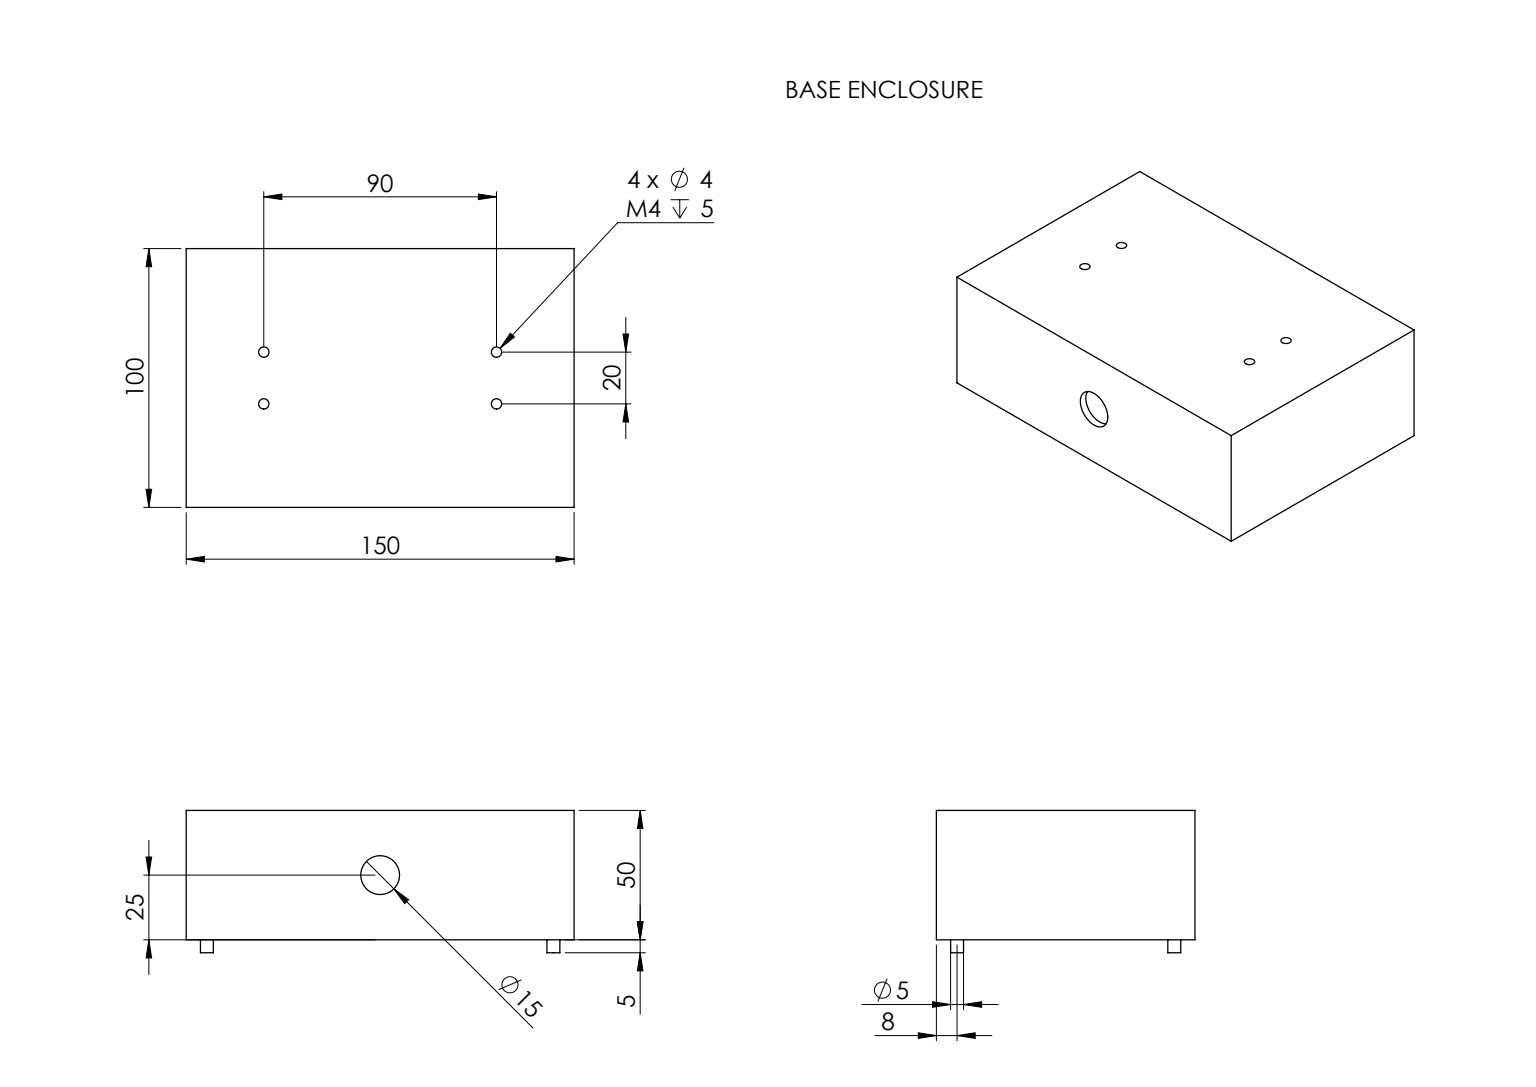
ISO-10303-21;
HEADER;
FILE_DESCRIPTION (('STEP AP214'),
    '1' );
FILE_NAME ('Base Enclosure^MAS-192.step',
    '2026-10-24T04:45:50',
    ( '' ),
    ( '' ),
    'SwSTEP 2.0',
    'SolidWorks 2026',
    '' );
FILE_SCHEMA (( 'AUTOMOTIVE_DESIGN' ));
ENDSEC;

DATA;
#4=ORIENTED_EDGE ( 'NONE', *, *, #1160, .F. ) ;
#11=FACE_OUTER_BOUND ( 'NONE', #1438, .T. ) ;
#19=CARTESIAN_POINT ( 'NONE',  ( 66.99999999999997158, -5.000000000000000000, -44.49999999999999289 ) ) ;
#24=EDGE_CURVE ( 'NONE', #3154, #2478, #414, .T. ) ;
#26=ORIENTED_EDGE ( 'NONE', *, *, #2595, .T. ) ;
#32=EDGE_CURVE ( 'NONE', #3203, #1539, #250, .T. ) ;
#35=VERTEX_POINT ( 'NONE', #2248 ) ;
#39=DIRECTION ( 'NONE',  ( -0.000000000000000000, 1.000000000000000000, -0.000000000000000000 ) ) ;
#41=ORIENTED_EDGE ( 'NONE', *, *, #2652, .T. ) ;
#43=EDGE_CURVE ( 'NONE', #2320, #2585, #1939, .T. ) ;
#48=FACE_OUTER_BOUND ( 'NONE', #483, .T. ) ;
#50=CYLINDRICAL_SURFACE ( 'NONE', #2706, 2.000000000000001776 ) ;
#51=CIRCLE ( 'NONE', #1902, 2.000000000000001776 ) ;
#55=AXIS2_PLACEMENT_3D ( 'NONE', #952, #3052, #3261 ) ;
#58=DIRECTION ( 'NONE',  ( -0.000000000000000000, 1.000000000000000000, -0.000000000000000000 ) ) ;
#62=CARTESIAN_POINT ( 'NONE',  ( 75.00000000000000000, 0.000000000000000000, 50.00000000000000000 ) ) ;
#65=CARTESIAN_POINT ( 'NONE',  ( 44.99999999999999289, 50.00000000000000000, -10.00000000000000533 ) ) ;
#66=PRODUCT_DEFINITION ( 'UNKNOWN', '', #1367, #996 ) ;
#70=ORIENTED_EDGE ( 'NONE', *, *, #2599, .T. ) ;
#72=LINE ( 'NONE', #1928, #2609 ) ;
#76=ADVANCED_FACE ( 'NONE', ( #408 ), #1739, .F. ) ;
#77=UNCERTAINTY_MEASURE_WITH_UNIT (LENGTH_MEASURE( 1.000000000000000082E-05 ), #1447, 'distance_accuracy_value', 'NONE');
#81=DIRECTION ( 'NONE',  ( 0.000000000000000000, 0.000000000000000000, -1.000000000000000000 ) ) ;
#82=LINE ( 'NONE', #1653, #2818 ) ;
#87=DIRECTION ( 'NONE',  ( 0.000000000000000000, 0.000000000000000000, 1.000000000000000000 ) ) ;
#88=ORIENTED_EDGE ( 'NONE', *, *, #1626, .T. ) ;
#92=DIRECTION ( 'NONE',  ( 0.000000000000000000, 0.000000000000000000, 1.000000000000000000 ) ) ;
#93=ADVANCED_FACE ( 'NONE', ( #3005 ), #3282, .F. ) ;
#94=CIRCLE ( 'NONE', #1191, 2.499999999999995115 ) ;
#96=CARTESIAN_POINT ( 'NONE',  ( -74.99999999999998579, 50.00000000000000000, -50.00000000000000000 ) ) ;
#97=AXIS2_PLACEMENT_3D ( 'NONE', #437, #2770, #128 ) ;
#103=FACE_BOUND ( 'NONE', #1561, .T. ) ;
#113=VERTEX_POINT ( 'NONE', #494 ) ;
#115=CARTESIAN_POINT ( 'NONE',  ( 66.99999999999997158, -5.000000000000000000, -39.50000000000000000 ) ) ;
#118=ADVANCED_FACE ( 'NONE', ( #1534 ), #3208, .F. ) ;
#119=CARTESIAN_POINT ( 'NONE',  ( -74.99999999999998579, 50.00000000000000000, -50.00000000000000000 ) ) ;
#121=VERTEX_POINT ( 'NONE', #1820 ) ;
#122=FACE_BOUND ( 'NONE', #2327, .T. ) ;
#123=FACE_OUTER_BOUND ( 'NONE', #1619, .T. ) ;
#125=LINE ( 'NONE', #3241, #2277 ) ;
#126=PRODUCT_CONTEXT ( 'NONE', #916, 'mechanical' ) ;
#128=DIRECTION ( 'NONE',  ( 1.000000000000000000, 0.000000000000000000, 0.000000000000000000 ) ) ;
#132=CARTESIAN_POINT ( 'NONE',  ( -66.99999999999997158, 0.000000000000000000, -41.99999999999999289 ) ) ;
#133=EDGE_CURVE ( 'NONE', #3190, #3154, #2535, .T. ) ;
#134=CARTESIAN_POINT ( 'NONE',  ( 0.000000000000000000, 25.00000000000000000, 50.00000000000000000 ) ) ;
#142=ORIENTED_EDGE ( 'NONE', *, *, #43, .F. ) ;
#148=DIRECTION ( 'NONE',  ( -0.000000000000000000, 1.000000000000000000, -0.000000000000000000 ) ) ;
#158=CIRCLE ( 'NONE', #2772, 2.499999999999995115 ) ;
#170=CARTESIAN_POINT ( 'NONE',  ( -75.00000000000000000, 50.00000000000000000, 50.00000000000000000 ) ) ;
#172=DIRECTION ( 'NONE',  ( 0.000000000000000000, 0.000000000000000000, -1.000000000000000000 ) ) ;
#173=EDGE_LOOP ( 'NONE', ( #2677, #3008, #1781, #962 ) ) ;
#176=ORIENTED_EDGE ( 'NONE', *, *, #433, .T. ) ;
#178=CARTESIAN_POINT ( 'NONE',  ( 44.99999999999999289, 50.00000000000000000, -12.00000000000000711 ) ) ;
#180=ORIENTED_EDGE ( 'NONE', *, *, #1149, .T. ) ;
#183=DIRECTION ( 'NONE',  ( -0.000000000000000000, 1.000000000000000000, -0.000000000000000000 ) ) ;
#185=DIRECTION ( 'NONE',  ( -0.000000000000000000, 1.000000000000000000, 0.000000000000000000 ) ) ;
#186=CARTESIAN_POINT ( 'NONE',  ( -66.99999999999997158, -5.000000000000000000, -41.99999999999999289 ) ) ;
#191=CARTESIAN_POINT ( 'NONE',  ( -45.00000000000000000, 43.79827876194489278, -9.999999999999994671 ) ) ;
#192=ORIENTED_EDGE ( 'NONE', *, *, #815, .F. ) ;
#203=ORIENTED_EDGE ( 'NONE', *, *, #133, .F. ) ;
#206=AXIS2_PLACEMENT_3D ( 'NONE', #944, #2253, #978 ) ;
#208=ORIENTED_EDGE ( 'NONE', *, *, #1510, .T. ) ;
#209=CIRCLE ( 'NONE', #2120, 2.499999999999995115 ) ;
#213=VECTOR ( 'NONE', #1718, 1000.000000000000000 ) ;
#226=ORIENTED_EDGE ( 'NONE', *, *, #721, .T. ) ;
#227=CARTESIAN_POINT ( 'NONE',  ( 7.500000000000000000, 25.00000000000000000, 50.00000000000000000 ) ) ;
#232=CARTESIAN_POINT ( 'NONE',  ( 45.00000000000000000, 50.00000000000000000, 9.999999999999994671 ) ) ;
#234=CARTESIAN_POINT ( 'NONE',  ( 66.99999999999997158, 0.000000000000000000, -41.99999999999999289 ) ) ;
#238=ORIENTED_EDGE ( 'NONE', *, *, #3134, .T. ) ;
#246=CARTESIAN_POINT ( 'NONE',  ( -44.99999999999999289, 45.00000000000000711, 12.00000000000000711 ) ) ;
#248=EDGE_CURVE ( 'NONE', #1538, #561, #458, .T. ) ;
#250=CIRCLE ( 'NONE', #2594, 2.000000000000001776 ) ;
#252=DIRECTION ( 'NONE',  ( 0.000000000000000000, 0.000000000000000000, 1.000000000000000000 ) ) ;
#263=AXIS2_PLACEMENT_3D ( 'NONE', #2360, #1555, #2633 ) ;
#264=ORIENTED_EDGE ( 'NONE', *, *, #1320, .T. ) ;
#267=DIRECTION ( 'NONE',  ( -0.000000000000000000, -1.000000000000000000, -0.000000000000000000 ) ) ;
#270=CYLINDRICAL_SURFACE ( 'NONE', #435, 2.000000000000001776 ) ;
#277=VERTEX_POINT ( 'NONE', #2558 ) ;
#279=AXIS2_PLACEMENT_3D ( 'NONE', #1513, #2605, #2846 ) ;
#282=DIRECTION ( 'NONE',  ( -1.000000000000000000, 0.000000000000000000, 0.000000000000000000 ) ) ;
#283=EDGE_CURVE ( 'NONE', #2585, #480, #1268, .T. ) ;
#286=CARTESIAN_POINT ( 'NONE',  ( 75.00000000000000000, 50.00000000000000000, 50.00000000000000000 ) ) ;
#290=DIRECTION ( 'NONE',  ( -0.000000000000000000, 1.000000000000000000, -0.000000000000000000 ) ) ;
#292=ORIENTED_EDGE ( 'NONE', *, *, #3182, .F. ) ;
#294=CYLINDRICAL_SURFACE ( 'NONE', #263, 2.000000000000001776 ) ;
#298=CYLINDRICAL_SURFACE ( 'NONE', #3325, 2.499999999999995115 ) ;
#300=DIRECTION ( 'NONE',  ( -0.000000000000000000, 1.000000000000000000, -0.000000000000000000 ) ) ;
#301=SURFACE_STYLE_USAGE ( .BOTH. , #1377 ) ;
#302=FACE_BOUND ( 'NONE', #1880, .T. ) ;
#307=ORIENTED_EDGE ( 'NONE', *, *, #2205, .T. ) ;
#308=LINE ( 'NONE', #1347, #2939 ) ;
#310=EDGE_CURVE ( 'NONE', #2398, #468, #2110, .T. ) ;
#314=AXIS2_PLACEMENT_3D ( 'NONE', #1704, #183, #1430 ) ;
#320=AXIS2_PLACEMENT_3D ( 'NONE', #3066, #1000, #486 ) ;
#323=CARTESIAN_POINT ( 'NONE',  ( 45.00000000000000000, 45.00000000000000711, 7.999999999999992895 ) ) ;
#324=VECTOR ( 'NONE', #1168, 999.9999999999998863 ) ;
#325=EDGE_CURVE ( 'NONE', #1539, #3203, #1947, .T. ) ;
#330=CYLINDRICAL_SURFACE ( 'NONE', #1898, 2.000000000000001776 ) ;
#332=LINE ( 'NONE', #2410, #1914 ) ;
#333=( LENGTH_UNIT ( ) NAMED_UNIT ( * ) SI_UNIT ( .MILLI., .METRE. ) );
#341=ORIENTED_EDGE ( 'NONE', *, *, #1510, .F. ) ;
#345=ORIENTED_EDGE ( 'NONE', *, *, #1998, .T. ) ;
#347=VERTEX_POINT ( 'NONE', #3209 ) ;
#350=DIRECTION ( 'NONE',  ( -0.000000000000000000, 1.000000000000000000, -0.000000000000000000 ) ) ;
#362=ADVANCED_FACE ( 'NONE', ( #830 ), #478, .F. ) ;
#368=DIRECTION ( 'NONE',  ( 0.000000000000000000, 0.000000000000000000, 1.000000000000000000 ) ) ;
#369=VECTOR ( 'NONE', #2367, 1000.000000000000000 ) ;
#372=ORIENTED_EDGE ( 'NONE', *, *, #3079, .F. ) ;
#375=CIRCLE ( 'NONE', #1306, 2.499999999999995115 ) ;
#376=ORIENTED_EDGE ( 'NONE', *, *, #1556, .T. ) ;
#377=FACE_BOUND ( 'NONE', #2636, .T. ) ;
#381=ORIENTED_EDGE ( 'NONE', *, *, #248, .F. ) ;
#382=CIRCLE ( 'NONE', #279, 2.499999999999995115 ) ;
#393=FACE_OUTER_BOUND ( 'NONE', #821, .T. ) ;
#400=ADVANCED_FACE ( 'NONE', ( #302, #1340 ), #2369, .F. ) ;
#402=ORIENTED_EDGE ( 'NONE', *, *, #3206, .F. ) ;
#403=CARTESIAN_POINT ( 'NONE',  ( 66.99999999999997158, -5.000000000000000000, -41.99999999999999289 ) ) ;
#407=CARTESIAN_POINT ( 'NONE',  ( -45.00000000000000000, 50.00000000000000000, -7.999999999999992895 ) ) ;
#408=FACE_OUTER_BOUND ( 'NONE', #1187, .T. ) ;
#411=ORIENTED_EDGE ( 'NONE', *, *, #2806, .T. ) ;
#414=CIRCLE ( 'NONE', #849, 7.500000000000000000 ) ;
#420=DIRECTION ( 'NONE',  ( 0.000000000000000000, -1.000000000000000000, 0.000000000000000000 ) ) ;
#421=CARTESIAN_POINT ( 'NONE',  ( -45.00000000000000000, 50.00000000000000000, -9.999999999999994671 ) ) ;
#423=DIRECTION ( 'NONE',  ( 0.000000000000000000, -1.000000000000000000, 0.000000000000000000 ) ) ;
#424=AXIS2_PLACEMENT_3D ( 'NONE', #2897, #2673, #1362 ) ;
#425=ADVANCED_FACE ( 'NONE', ( #48 ), #847, .T. ) ;
#426=( NAMED_UNIT ( * ) SI_UNIT ( $, .STERADIAN. ) SOLID_ANGLE_UNIT ( ) );
#427=AXIS2_PLACEMENT_3D ( 'NONE', #2477, #1108, #87 ) ;
#429=ORIENTED_EDGE ( 'NONE', *, *, #1320, .F. ) ;
#432=VECTOR ( 'NONE', #2012, 999.9999999999998863 ) ;
#433=EDGE_CURVE ( 'NONE', #2761, #2259, #1907, .T. ) ;
#435=AXIS2_PLACEMENT_3D ( 'NONE', #232, #1280, #3107 ) ;
#437=CARTESIAN_POINT ( 'NONE',  ( 0.000000000000000000, 25.00000000000000000, 47.00000000000000000 ) ) ;
#443=EDGE_CURVE ( 'NONE', #277, #2259, #3036, .T. ) ;
#444=DIRECTION ( 'NONE',  ( -0.000000000000000000, 1.000000000000000000, -0.000000000000000000 ) ) ;
#448=VERTEX_POINT ( 'NONE', #2198 ) ;
#453=PLANE ( 'NONE',  #2663 ) ;
#454=ORIENTED_EDGE ( 'NONE', *, *, #1869, .T. ) ;
#458=LINE ( 'NONE', #1514, #910 ) ;
#460=LINE ( 'NONE', #3299, #3221 ) ;
#461=ORIENTED_EDGE ( 'NONE', *, *, #1991, .F. ) ;
#463=CARTESIAN_POINT ( 'NONE',  ( -66.99999999999997158, -5.000000000000000000, 39.50000000000000000 ) ) ;
#466=PLANE ( 'NONE',  #320 ) ;
#468=VERTEX_POINT ( 'NONE', #1178 ) ;
#470=DIRECTION ( 'NONE',  ( 1.049727191138620668E-16, 0.5150380749100514910, -0.8571673007021138879 ) ) ;
#473=CARTESIAN_POINT ( 'NONE',  ( -45.00000000000000000, 50.00000000000000000, -9.999999999999994671 ) ) ;
#478=CONICAL_SURFACE ( 'NONE', #424, 2.000000000000001776, 1.029744258676657642 ) ;
#479=ADVANCED_BREP_SHAPE_REPRESENTATION ( '', ( #2792, #3111 ), #1204 ) ;
#480=VERTEX_POINT ( 'NONE', #2212 ) ;
#483=EDGE_LOOP ( 'NONE', ( #402, #2152, #70, #1488 ) ) ;
#486=DIRECTION ( 'NONE',  ( 0.000000000000000000, -0.000000000000000000, -1.000000000000000000 ) ) ;
#492=ADVANCED_FACE ( 'NONE', ( #3247 ), #1936, .F. ) ;
#494=CARTESIAN_POINT ( 'NONE',  ( 44.99999999999999289, 45.00000000000000711, -8.000000000000003553 ) ) ;
#495=CARTESIAN_POINT ( 'NONE',  ( 75.00000000000000000, 0.000000000000000000, -50.00000000000000000 ) ) ;
#498=ORIENTED_EDGE ( 'NONE', *, *, #1764, .F. ) ;
#499=VERTEX_POINT ( 'NONE', #1703 ) ;
#504=DIRECTION ( 'NONE',  ( 0.000000000000000000, 0.000000000000000000, 1.000000000000000000 ) ) ;
#507=FACE_OUTER_BOUND ( 'NONE', #752, .T. ) ;
#510=PRODUCT ( 'Base Enclosure^MAS-192', 'Base Enclosure^MAS-192', '', ( #126 ) ) ;
#511=EDGE_CURVE ( 'NONE', #1605, #1554, #94, .T. ) ;
#515=EDGE_LOOP ( 'NONE', ( #3254, #1310, #3355, #3169 ) ) ;
#520=DIRECTION ( 'NONE',  ( -0.000000000000000000, 1.000000000000000000, -0.000000000000000000 ) ) ;
#523=LINE ( 'NONE', #2574, #1629 ) ;
#531=VERTEX_POINT ( 'NONE', #2484 ) ;
#532=AXIS2_PLACEMENT_3D ( 'NONE', #403, #2962, #671 ) ;
#537=CIRCLE ( 'NONE', #3045, 2.000000000000001776 ) ;
#548=ORIENTED_EDGE ( 'NONE', *, *, #3058, .T. ) ;
#551=ORIENTED_EDGE ( 'NONE', *, *, #1747, .F. ) ;
#552=DIRECTION ( 'NONE',  ( 0.000000000000000000, 0.000000000000000000, 1.000000000000000000 ) ) ;
#553=UNCERTAINTY_MEASURE_WITH_UNIT (LENGTH_MEASURE( 1.000000000000000082E-05 ), #1906, 'distance_accuracy_value', 'NONE');
#557=CARTESIAN_POINT ( 'NONE',  ( 45.00000000000000000, 45.00000000000000711, 9.999999999999994671 ) ) ;
#561=VERTEX_POINT ( 'NONE', #1479 ) ;
#562=ORIENTED_EDGE ( 'NONE', *, *, #1667, .F. ) ;
#564=ORIENTED_EDGE ( 'NONE', *, *, #2324, .F. ) ;
#569=DIRECTION ( 'NONE',  ( -0.000000000000000000, 1.000000000000000000, -0.000000000000000000 ) ) ;
#577=FACE_OUTER_BOUND ( 'NONE', #3185, .T. ) ;
#584=AXIS2_PLACEMENT_3D ( 'NONE', #1266, #520, #989 ) ;
#590=DIRECTION ( 'NONE',  ( 0.000000000000000000, 0.000000000000000000, 1.000000000000000000 ) ) ;
#594=VERTEX_POINT ( 'NONE', #2044 ) ;
#597=CARTESIAN_POINT ( 'NONE',  ( -44.99999999999999289, 45.00000000000000711, 10.00000000000000533 ) ) ;
#598=DIRECTION ( 'NONE',  ( 1.000000000000000000, -0.000000000000000000, 1.387778780781445676E-16 ) ) ;
#603=EDGE_CURVE ( 'NONE', #448, #2691, #764, .T. ) ;
#609=ORIENTED_EDGE ( 'NONE', *, *, #721, .F. ) ;
#611=EDGE_CURVE ( 'NONE', #2086, #347, #1767, .T. ) ;
#618=CARTESIAN_POINT ( 'NONE',  ( -45.00000000000000000, 50.00000000000000000, -11.99999999999999645 ) ) ;
#620=PRESENTATION_STYLE_ASSIGNMENT (( #301 ) ) ;
#623=FACE_OUTER_BOUND ( 'NONE', #2591, .T. ) ;
#626=DIRECTION ( 'NONE',  ( -0.000000000000000000, 1.000000000000000000, -0.000000000000000000 ) ) ;
#630=EDGE_CURVE ( 'NONE', #347, #2291, #3348, .T. ) ;
#633=ADVANCED_FACE ( 'NONE', ( #781 ), #2027, .F. ) ;
#642=CARTESIAN_POINT ( 'NONE',  ( -66.99999999999997158, -5.000000000000000000, 44.49999999999999289 ) ) ;
#645=DIRECTION ( 'NONE',  ( -0.000000000000000000, 1.000000000000000000, -0.000000000000000000 ) ) ;
#646=EDGE_CURVE ( 'NONE', #2761, #113, #2061, .T. ) ;
#651=EDGE_LOOP ( 'NONE', ( #1357, #2209 ) ) ;
#655=ORIENTED_EDGE ( 'NONE', *, *, #3079, .T. ) ;
#656=CARTESIAN_POINT ( 'NONE',  ( 44.99999999999999289, 45.00000000000000711, -12.00000000000000711 ) ) ;
#657=DIRECTION ( 'NONE',  ( 0.000000000000000000, 0.000000000000000000, 1.000000000000000000 ) ) ;
#660=DIRECTION ( 'NONE',  ( 1.000000000000000000, 0.000000000000000000, 0.000000000000000000 ) ) ;
#661=CYLINDRICAL_SURFACE ( 'NONE', #314, 2.499999999999995115 ) ;
#663=DIRECTION ( 'NONE',  ( 0.000000000000000000, 0.000000000000000000, 1.000000000000000000 ) ) ;
#671=DIRECTION ( 'NONE',  ( 0.000000000000000000, -0.000000000000000000, -1.000000000000000000 ) ) ;
#672=CARTESIAN_POINT ( 'NONE',  ( 66.99999999999997158, -5.000000000000000000, -41.99999999999999289 ) ) ;
#673=FACE_OUTER_BOUND ( 'NONE', #3258, .T. ) ;
#678=( NAMED_UNIT ( * ) PLANE_ANGLE_UNIT ( ) SI_UNIT ( $, .RADIAN. ) );
#679=ORIENTED_EDGE ( 'NONE', *, *, #3237, .T. ) ;
#685=SHAPE_REPRESENTATION ( 'Base Enclosure^MAS-192', ( #3111 ), #1204 ) ;
#690=CARTESIAN_POINT ( 'NONE',  ( -7.500000000000000000, 25.00000000000000000, 47.00000000000000000 ) ) ;
#695=AXIS2_PLACEMENT_3D ( 'NONE', #1058, #2991, #2351 ) ;
#696=DIRECTION ( 'NONE',  ( 0.000000000000000000, 0.000000000000000000, 1.000000000000000000 ) ) ;
#700=DIRECTION ( 'NONE',  ( -0.000000000000000000, 1.000000000000000000, 0.000000000000000000 ) ) ;
#702=CIRCLE ( 'NONE', #1036, 2.499999999999995115 ) ;
#709=ORIENTED_EDGE ( 'NONE', *, *, #2219, .T. ) ;
#719=VERTEX_POINT ( 'NONE', #2682 ) ;
#721=EDGE_CURVE ( 'NONE', #468, #3203, #2942, .T. ) ;
#728=LINE ( 'NONE', #1509, #1455 ) ;
#731=CARTESIAN_POINT ( 'NONE',  ( -66.99999999999997158, 0.000000000000000000, 41.99999999999999289 ) ) ;
#733=ORIENTED_EDGE ( 'NONE', *, *, #3213, .T. ) ;
#735=ORIENTED_EDGE ( 'NONE', *, *, #2411, .F. ) ;
#737=DIRECTION ( 'NONE',  ( 0.000000000000000000, -1.000000000000000000, 0.000000000000000000 ) ) ;
#748=ORIENTED_EDGE ( 'NONE', *, *, #283, .T. ) ;
#752=EDGE_LOOP ( 'NONE', ( #2089, #1877, #2801, #609 ) ) ;
#757=AXIS2_PLACEMENT_3D ( 'NONE', #1609, #2090, #2144 ) ;
#758=CIRCLE ( 'NONE', #2664, 2.499999999999995115 ) ;
#763=ORIENTED_EDGE ( 'NONE', *, *, #1960, .F. ) ;
#764=LINE ( 'NONE', #2586, #2546 ) ;
#768=CARTESIAN_POINT ( 'NONE',  ( -45.00000000000000000, 45.00000000000000711, -9.999999999999994671 ) ) ;
#771=PLANE ( 'NONE',  #2227 ) ;
#774=VERTEX_POINT ( 'NONE', #2712 ) ;
#777=EDGE_CURVE ( 'NONE', #3174, #895, #2769, .T. ) ;
#781=FACE_OUTER_BOUND ( 'NONE', #515, .T. ) ;
#791=EDGE_LOOP ( 'NONE', ( #1449, #2166, #1868, #3198 ) ) ;
#792=LINE ( 'NONE', #1337, #2392 ) ;
#798=CARTESIAN_POINT ( 'NONE',  ( 0.000000000000000000, 25.00000000000000000, 47.00000000000000000 ) ) ;
#801=VERTEX_POINT ( 'NONE', #857 ) ;
#805=AXIS2_PLACEMENT_3D ( 'NONE', #2415, #865, #2687 ) ;
#806=ORIENTED_EDGE ( 'NONE', *, *, #2411, .T. ) ;
#809=CIRCLE ( 'NONE', #2548, 2.000000000000001776 ) ;
#811=AXIS2_PLACEMENT_3D ( 'NONE', #2678, #2903, #1154 ) ;
#812=ORIENTED_EDGE ( 'NONE', *, *, #2257, .F. ) ;
#813=FACE_OUTER_BOUND ( 'NONE', #173, .T. ) ;
#815=EDGE_CURVE ( 'NONE', #561, #719, #125, .T. ) ;
#817=CARTESIAN_POINT ( 'NONE',  ( 75.00000000000000000, 50.00000000000000000, 50.00000000000000000 ) ) ;
#818=DIRECTION ( 'NONE',  ( 0.000000000000000000, 0.000000000000000000, 1.000000000000000000 ) ) ;
#821=EDGE_LOOP ( 'NONE', ( #1255, #1521, #1611, #3308 ) ) ;
#824=VERTEX_POINT ( 'NONE', #1932 ) ;
#826=CYLINDRICAL_SURFACE ( 'NONE', #3105, 2.499999999999995115 ) ;
#828=ORIENTED_EDGE ( 'NONE', *, *, #1481, .T. ) ;
#830=FACE_OUTER_BOUND ( 'NONE', #2341, .T. ) ;
#832=DIRECTION ( 'NONE',  ( -0.000000000000000000, 1.000000000000000000, -0.000000000000000000 ) ) ;
#835=ORIENTED_EDGE ( 'NONE', *, *, #511, .F. ) ;
#837=FACE_OUTER_BOUND ( 'NONE', #1826, .T. ) ;
#842=EDGE_CURVE ( 'NONE', #1605, #1570, #332, .T. ) ;
#847=CYLINDRICAL_SURFACE ( 'NONE', #805, 2.499999999999995115 ) ;
#848=CARTESIAN_POINT ( 'NONE',  ( -45.00000000000000000, 50.00000000000000000, -9.999999999999994671 ) ) ;
#849=AXIS2_PLACEMENT_3D ( 'NONE', #134, #663, #1707 ) ;
#857=CARTESIAN_POINT ( 'NONE',  ( -44.99999999999999289, 50.00000000000000000, 8.000000000000003553 ) ) ;
#861=AXIS2_PLACEMENT_3D ( 'NONE', #1652, #290, #1635 ) ;
#864=SURFACE_STYLE_FILL_AREA ( #3179 ) ;
#865=DIRECTION ( 'NONE',  ( -0.000000000000000000, 1.000000000000000000, -0.000000000000000000 ) ) ;
#875=DIRECTION ( 'NONE',  ( 0.000000000000000000, 0.000000000000000000, 1.000000000000000000 ) ) ;
#876=DIRECTION ( 'NONE',  ( 0.000000000000000000, 0.5150380749100514910, 0.8571673007021138879 ) ) ;
#883=DIRECTION ( 'NONE',  ( -0.000000000000000000, -0.000000000000000000, 1.000000000000000000 ) ) ;
#884=DIRECTION ( 'NONE',  ( -0.000000000000000000, 1.000000000000000000, -0.000000000000000000 ) ) ;
#888=ORIENTED_EDGE ( 'NONE', *, *, #2262, .T. ) ;
#891=EDGE_CURVE ( 'NONE', #1277, #3215, #1450, .T. ) ;
#893=DIRECTION ( 'NONE',  ( -0.000000000000000000, 1.000000000000000000, -0.000000000000000000 ) ) ;
#895=VERTEX_POINT ( 'NONE', #463 ) ;
#910=VECTOR ( 'NONE', #1496, 1000.000000000000000 ) ;
#913=AXIS2_PLACEMENT_3D ( 'NONE', #3141, #2879, #1165 ) ;
#916=APPLICATION_CONTEXT ( 'automotive_design' ) ;
#917=CIRCLE ( 'NONE', #1141, 7.500000000000000000 ) ;
#921=VECTOR ( 'NONE', #3175, 1000.000000000000000 ) ;
#933=ORIENTED_EDGE ( 'NONE', *, *, #283, .F. ) ;
#937=CARTESIAN_POINT ( 'NONE',  ( 0.000000000000000000, 25.00000000000000000, 47.00000000000000000 ) ) ;
#939=DIRECTION ( 'NONE',  ( -0.000000000000000000, 1.000000000000000000, -0.000000000000000000 ) ) ;
#944=CARTESIAN_POINT ( 'NONE',  ( 66.99999999999997158, -5.000000000000000000, 41.99999999999999289 ) ) ;
#950=ORIENTED_EDGE ( 'NONE', *, *, #1226, .F. ) ;
#951=DIRECTION ( 'NONE',  ( 0.000000000000000000, -1.000000000000000000, 0.000000000000000000 ) ) ;
#952=CARTESIAN_POINT ( 'NONE',  ( 66.99999999999997158, 0.000000000000000000, 41.99999999999999289 ) ) ;
#953=ADVANCED_FACE ( 'NONE', ( #2745 ), #2269, .T. ) ;
#954=LINE ( 'NONE', #1988, #1308 ) ;
#956=CARTESIAN_POINT ( 'NONE',  ( 45.00000000000000000, 45.00000000000000711, 7.999999999999992895 ) ) ;
#962=ORIENTED_EDGE ( 'NONE', *, *, #1226, .T. ) ;
#965=AXIS2_PLACEMENT_3D ( 'NONE', #3127, #3072, #1786 ) ;
#968=LINE ( 'NONE', #2315, #981 ) ;
#970=EDGE_CURVE ( 'NONE', #2106, #1968, #809, .T. ) ;
#978=DIRECTION ( 'NONE',  ( 0.000000000000000000, 0.000000000000000000, 1.000000000000000000 ) ) ;
#980=CIRCLE ( 'NONE', #2557, 2.499999999999995115 ) ;
#981=VECTOR ( 'NONE', #1533, 1000.000000000000000 ) ;
#982=EDGE_LOOP ( 'NONE', ( #2278, #548, #2419 ) ) ;
#984=FACE_BOUND ( 'NONE', #1823, .T. ) ;
#989=DIRECTION ( 'NONE',  ( 0.000000000000000000, 0.000000000000000000, 1.000000000000000000 ) ) ;
#991=FACE_OUTER_BOUND ( 'NONE', #1558, .T. ) ;
#992=ADVANCED_FACE ( 'NONE', ( #1471 ), #3303, .F. ) ;
#996=PRODUCT_DEFINITION_CONTEXT ( 'detailed design', #2030, 'design' ) ;
#999=ORIENTED_EDGE ( 'NONE', *, *, #24, .F. ) ;
#1000=DIRECTION ( 'NONE',  ( 0.000000000000000000, -1.000000000000000000, 0.000000000000000000 ) ) ;
#1004=ADVANCED_FACE ( 'NONE', ( #3132 ), #294, .F. ) ;
#1007=DIRECTION ( 'NONE',  ( 0.000000000000000000, 0.000000000000000000, 1.000000000000000000 ) ) ;
#1010=ORIENTED_EDGE ( 'NONE', *, *, #2997, .F. ) ;
#1025=ORIENTED_EDGE ( 'NONE', *, *, #2262, .F. ) ;
#1026=VECTOR ( 'NONE', #1683, 1000.000000000000000 ) ;
#1027=VECTOR ( 'NONE', #876, 999.9999999999998863 ) ;
#1036=AXIS2_PLACEMENT_3D ( 'NONE', #186, #423, #3006 ) ;
#1038=UNCERTAINTY_MEASURE_WITH_UNIT (LENGTH_MEASURE( 1.000000000000000082E-05 ), #333, 'distance_accuracy_value', 'NONE');
#1046=DIRECTION ( 'NONE',  ( -0.000000000000000000, 1.000000000000000000, -0.000000000000000000 ) ) ;
#1055=CARTESIAN_POINT ( 'NONE',  ( 75.00000000000000000, 50.00000000000000000, 50.00000000000000000 ) ) ;
#1058=CARTESIAN_POINT ( 'NONE',  ( -66.99999999999997158, -5.000000000000000000, 41.99999999999999289 ) ) ;
#1069=DIRECTION ( 'NONE',  ( 0.000000000000000000, 0.000000000000000000, -1.000000000000000000 ) ) ;
#1078=LINE ( 'NONE', #2111, #2438 ) ;
#1086=VECTOR ( 'NONE', #1803, 1000.000000000000000 ) ;
#1093=CIRCLE ( 'NONE', #2992, 2.499999999999995115 ) ;
#1100=DIRECTION ( 'NONE',  ( -0.000000000000000000, 1.000000000000000000, -0.000000000000000000 ) ) ;
#1104=ORIENTED_EDGE ( 'NONE', *, *, #2997, .T. ) ;
#1106=DIRECTION ( 'NONE',  ( 0.000000000000000000, 0.000000000000000000, 1.000000000000000000 ) ) ;
#1108=DIRECTION ( 'NONE',  ( -0.000000000000000000, 1.000000000000000000, -0.000000000000000000 ) ) ;
#1109=ORIENTED_EDGE ( 'NONE', *, *, #2475, .F. ) ;
#1110=CARTESIAN_POINT ( 'NONE',  ( 66.99999999999997158, -5.000000000000000000, 41.99999999999999289 ) ) ;
#1113=ORIENTED_EDGE ( 'NONE', *, *, #2350, .F. ) ;
#1114=CARTESIAN_POINT ( 'NONE',  ( -44.99999999999999289, 50.00000000000000000, 10.00000000000000533 ) ) ;
#1117=FACE_OUTER_BOUND ( 'NONE', #791, .T. ) ;
#1119=LINE ( 'NONE', #1150, #2339 ) ;
#1129=SHAPE_REPRESENTATION_RELATIONSHIP ( 'NONE' , 'NONE' ,  #685, #479 ) ;
#1130=CARTESIAN_POINT ( 'NONE',  ( 45.00000000000000000, 45.00000000000000711, 11.99999999999999645 ) ) ;
#1133=ORIENTED_EDGE ( 'NONE', *, *, #777, .T. ) ;
#1135=ORIENTED_EDGE ( 'NONE', *, *, #611, .T. ) ;
#1137=DIRECTION ( 'NONE',  ( -0.000000000000000000, 1.000000000000000000, -0.000000000000000000 ) ) ;
#1139=DIRECTION ( 'NONE',  ( -0.000000000000000000, 1.000000000000000000, -0.000000000000000000 ) ) ;
#1140=ORIENTED_EDGE ( 'NONE', *, *, #443, .T. ) ;
#1141=AXIS2_PLACEMENT_3D ( 'NONE', #1375, #92, #1884 ) ;
#1149=EDGE_CURVE ( 'NONE', #1763, #1570, #375, .T. ) ;
#1150=CARTESIAN_POINT ( 'NONE',  ( -75.00000000000000000, 50.00000000000000000, 50.00000000000000000 ) ) ;
#1151=CIRCLE ( 'NONE', #2617, 2.499999999999995115 ) ;
#1152=EDGE_LOOP ( 'NONE', ( #2290, #341, #2481, #2578 ) ) ;
#1153=ORIENTED_EDGE ( 'NONE', *, *, #2802, .T. ) ;
#1154=DIRECTION ( 'NONE',  ( 0.000000000000000000, -0.000000000000000000, -1.000000000000000000 ) ) ;
#1160=EDGE_CURVE ( 'NONE', #2976, #1539, #72, .T. ) ;
#1165=DIRECTION ( 'NONE',  ( 0.000000000000000000, 0.000000000000000000, 1.000000000000000000 ) ) ;
#1166=CARTESIAN_POINT ( 'NONE',  ( -45.00000000000000000, 45.00000000000000711, -7.999999999999992895 ) ) ;
#1168=DIRECTION ( 'NONE',  ( 1.049727191138620668E-16, 0.5150380749100514910, -0.8571673007021138879 ) ) ;
#1172=DIRECTION ( 'NONE',  ( 0.000000000000000000, 0.000000000000000000, -1.000000000000000000 ) ) ;
#1173=DIRECTION ( 'NONE',  ( 0.000000000000000000, 0.000000000000000000, 1.000000000000000000 ) ) ;
#1174=ORIENTED_EDGE ( 'NONE', *, *, #1747, .T. ) ;
#1177=CYLINDRICAL_SURFACE ( 'NONE', #2116, 2.499999999999995115 ) ;
#1178=CARTESIAN_POINT ( 'NONE',  ( 45.00000000000000000, 45.00000000000000711, 11.99999999999999645 ) ) ;
#1179=CARTESIAN_POINT ( 'NONE',  ( 66.99999999999997158, 0.000000000000000000, 41.99999999999999289 ) ) ;
#1183=CARTESIAN_POINT ( 'NONE',  ( 44.99999999999999289, 45.00000000000000711, -12.00000000000000711 ) ) ;
#1184=ORIENTED_EDGE ( 'NONE', *, *, #2784, .T. ) ;
#1187=EDGE_LOOP ( 'NONE', ( #806, #2969 ) ) ;
#1188=FACE_OUTER_BOUND ( 'NONE', #2799, .T. ) ;
#1190=AXIS2_PLACEMENT_3D ( 'NONE', #2752, #2724, #2230 ) ;
#1191=AXIS2_PLACEMENT_3D ( 'NONE', #672, #951, #1412 ) ;
#1194=AXIS2_PLACEMENT_3D ( 'NONE', #2910, #569, #1983 ) ;
#1197=VECTOR ( 'NONE', #1069, 1000.000000000000000 ) ;
#1198=CIRCLE ( 'NONE', #3106, 2.000000000000001776 ) ;
#1199=DIRECTION ( 'NONE',  ( -0.000000000000000000, 1.000000000000000000, -0.000000000000000000 ) ) ;
#1201=CIRCLE ( 'NONE', #2613, 2.499999999999995115 ) ;
#1204=( GEOMETRIC_REPRESENTATION_CONTEXT ( 3 ) GLOBAL_UNCERTAINTY_ASSIGNED_CONTEXT ( ( #1038 ) ) GLOBAL_UNIT_ASSIGNED_CONTEXT ( ( #333, #1819, #2430 ) ) REPRESENTATION_CONTEXT ( 'NONE', 'WORKASPACE' ) );
#1205=DIRECTION ( 'NONE',  ( 0.000000000000000000, 0.000000000000000000, 1.000000000000000000 ) ) ;
#1216=CARTESIAN_POINT ( 'NONE',  ( -66.99999999999997158, -5.000000000000000000, 39.50000000000000000 ) ) ;
#1218=ADVANCED_FACE ( 'NONE', ( #2439 ), #1576, .F. ) ;
#1220=DIRECTION ( 'NONE',  ( 1.049727191138620668E-16, 0.5150380749100514910, -0.8571673007021138879 ) ) ;
#1226=EDGE_CURVE ( 'NONE', #2291, #801, #51, .T. ) ;
#1233=ADVANCED_FACE ( 'NONE', ( #122, #103, #377, #1642, #577 ), #1864, .T. ) ;
#1241=CARTESIAN_POINT ( 'NONE',  ( -44.99999999999999289, 50.00000000000000000, 12.00000000000000711 ) ) ;
#1246=CARTESIAN_POINT ( 'NONE',  ( -66.99999999999997158, -5.000000000000000000, -41.99999999999999289 ) ) ;
#1250=EDGE_CURVE ( 'NONE', #2460, #1968, #308, .T. ) ;
#1251=DIRECTION ( 'NONE',  ( 0.000000000000000000, -1.000000000000000000, 0.000000000000000000 ) ) ;
#1252=CIRCLE ( 'NONE', #3161, 2.499999999999995115 ) ;
#1255=ORIENTED_EDGE ( 'NONE', *, *, #1304, .F. ) ;
#1257=AXIS2_PLACEMENT_3D ( 'NONE', #3233, #884, #818 ) ;
#1265=EDGE_LOOP ( 'NONE', ( #1109, #1927 ) ) ;
#1266=CARTESIAN_POINT ( 'NONE',  ( 44.99999999999999289, 45.00000000000000711, -10.00000000000000533 ) ) ;
#1268=LINE ( 'NONE', #817, #2058 ) ;
#1275=DIRECTION ( 'NONE',  ( 0.000000000000000000, 0.000000000000000000, 1.000000000000000000 ) ) ;
#1277=VERTEX_POINT ( 'NONE', #3219 ) ;
#1280=DIRECTION ( 'NONE',  ( -0.000000000000000000, 1.000000000000000000, -0.000000000000000000 ) ) ;
#1282=CARTESIAN_POINT ( 'NONE',  ( 66.99999999999997158, 0.000000000000000000, -44.49999999999999289 ) ) ;
#1288=EDGE_CURVE ( 'NONE', #801, #2291, #537, .T. ) ;
#1296=CARTESIAN_POINT ( 'NONE',  ( 45.00000000000000000, 45.00000000000000711, 9.999999999999994671 ) ) ;
#1300=CIRCLE ( 'NONE', #2446, 2.499999999999995115 ) ;
#1304=EDGE_CURVE ( 'NONE', #448, #2972, #702, .T. ) ;
#1306=AXIS2_PLACEMENT_3D ( 'NONE', #1915, #2391, #1172 ) ;
#1308=VECTOR ( 'NONE', #444, 1000.000000000000000 ) ;
#1310=ORIENTED_EDGE ( 'NONE', *, *, #133, .T. ) ;
#1319=VERTEX_POINT ( 'NONE', #2476 ) ;
#1320=EDGE_CURVE ( 'NONE', #2398, #2976, #1694, .T. ) ;
#1321=ORIENTED_EDGE ( 'NONE', *, *, #1727, .T. ) ;
#1324=LINE ( 'NONE', #62, #1197 ) ;
#1326=ORIENTED_EDGE ( 'NONE', *, *, #970, .F. ) ;
#1327=CYLINDRICAL_SURFACE ( 'NONE', #2001, 2.000000000000001776 ) ;
#1333=PLANE ( 'NONE',  #1901 ) ;
#1337=CARTESIAN_POINT ( 'NONE',  ( -44.99999999999999289, 50.00000000000000000, 8.000000000000003553 ) ) ;
#1340=FACE_OUTER_BOUND ( 'NONE', #1529, .T. ) ;
#1343=CARTESIAN_POINT ( 'NONE',  ( 66.99999999999997158, -5.000000000000000000, -41.99999999999999289 ) ) ;
#1344=ORIENTED_EDGE ( 'NONE', *, *, #1991, .T. ) ;
#1347=CARTESIAN_POINT ( 'NONE',  ( -45.00000000000000000, 45.00000000000000711, -7.999999999999992895 ) ) ;
#1349=AXIS2_PLACEMENT_3D ( 'NONE', #1179, #3296, #1937 ) ;
#1352=DIRECTION ( 'NONE',  ( -0.000000000000000000, 1.000000000000000000, -0.000000000000000000 ) ) ;
#1353=AXIS2_PLACEMENT_3D ( 'NONE', #3038, #700, #2019 ) ;
#1356=CONICAL_SURFACE ( 'NONE', #3163, 2.000000000000001776, 1.029744258676657642 ) ;
#1357=ORIENTED_EDGE ( 'NONE', *, *, #32, .F. ) ;
#1359=CARTESIAN_POINT ( 'NONE',  ( -44.99999999999999289, 45.00000000000000711, 8.000000000000003553 ) ) ;
#1362=DIRECTION ( 'NONE',  ( 0.000000000000000000, 0.000000000000000000, 1.000000000000000000 ) ) ;
#1367=PRODUCT_DEFINITION_FORMATION_WITH_SPECIFIED_SOURCE ( 'ANY', '', #510, .NOT_KNOWN. ) ;
#1371=ORIENTED_EDGE ( 'NONE', *, *, #1970, .T. ) ;
#1374=ORIENTED_EDGE ( 'NONE', *, *, #1970, .F. ) ;
#1375=CARTESIAN_POINT ( 'NONE',  ( 0.000000000000000000, 25.00000000000000000, 47.00000000000000000 ) ) ;
#1377=SURFACE_SIDE_STYLE ('',( #864 ) ) ;
#1379=DIRECTION ( 'NONE',  ( -0.000000000000000000, -1.000000000000000000, -0.000000000000000000 ) ) ;
#1381=ORIENTED_EDGE ( 'NONE', *, *, #1551, .T. ) ;
#1391=DIRECTION ( 'NONE',  ( -0.000000000000000000, 1.000000000000000000, -0.000000000000000000 ) ) ;
#1393=CARTESIAN_POINT ( 'NONE',  ( 66.99999999999997158, 0.000000000000000000, -39.50000000000000000 ) ) ;
#1398=DIRECTION ( 'NONE',  ( -0.000000000000000000, 1.000000000000000000, -0.000000000000000000 ) ) ;
#1403=VECTOR ( 'NONE', #470, 999.9999999999998863 ) ;
#1408=CARTESIAN_POINT ( 'NONE',  ( -75.00000000000000000, 50.00000000000000000, 50.00000000000000000 ) ) ;
#1411=EDGE_CURVE ( 'NONE', #480, #774, #460, .T. ) ;
#1412=DIRECTION ( 'NONE',  ( 0.000000000000000000, 0.000000000000000000, -1.000000000000000000 ) ) ;
#1416=MECHANICAL_DESIGN_GEOMETRIC_PRESENTATION_REPRESENTATION('',(#1905),#2128);
#1417=ORIENTED_EDGE ( 'NONE', *, *, #2205, .F. ) ;
#1421=DIRECTION ( 'NONE',  ( 0.000000000000000000, 0.000000000000000000, 1.000000000000000000 ) ) ;
#1425=CARTESIAN_POINT ( 'NONE',  ( 45.00000000000000000, 50.00000000000000000, 11.99999999999999645 ) ) ;
#1430=DIRECTION ( 'NONE',  ( 0.000000000000000000, 0.000000000000000000, 1.000000000000000000 ) ) ;
#1438=EDGE_LOOP ( 'NONE', ( #2817, #733, #2600, #2268 ) ) ;
#1439=CARTESIAN_POINT ( 'NONE',  ( -44.99999999999999289, 50.00000000000000000, 12.00000000000000711 ) ) ;
#1447=( LENGTH_UNIT ( ) NAMED_UNIT ( * ) SI_UNIT ( .MILLI., .METRE. ) );
#1449=ORIENTED_EDGE ( 'NONE', *, *, #1779, .F. ) ;
#1450=LINE ( 'NONE', #1487, #2443 ) ;
#1453=LINE ( 'NONE', #618, #1026 ) ;
#1454=AXIS2_PLACEMENT_3D ( 'NONE', #2983, #185, #1483 ) ;
#1455=VECTOR ( 'NONE', #267, 1000.000000000000000 ) ;
#1456=ADVANCED_FACE ( 'NONE', ( #991 ), #1356, .F. ) ;
#1459=PRODUCT_DEFINITION_SHAPE ( 'NONE', 'NONE',  #66 ) ;
#1462=DIRECTION ( 'NONE',  ( 0.000000000000000000, 0.000000000000000000, 1.000000000000000000 ) ) ;
#1471=FACE_OUTER_BOUND ( 'NONE', #1724, .T. ) ;
#1478=ORIENTED_EDGE ( 'NONE', *, *, #1551, .F. ) ;
#1479=CARTESIAN_POINT ( 'NONE',  ( -74.99999999999998579, 0.000000000000000000, -50.00000000000000000 ) ) ;
#1481=EDGE_CURVE ( 'NONE', #499, #3078, #1093, .T. ) ;
#1482=CARTESIAN_POINT ( 'NONE',  ( 66.99999999999997158, 0.000000000000000000, 44.49999999999999289 ) ) ;
#1483=DIRECTION ( 'NONE',  ( 0.000000000000000000, 0.000000000000000000, 1.000000000000000000 ) ) ;
#1485=CARTESIAN_POINT ( 'NONE',  ( -66.99999999999997158, -5.000000000000000000, 41.99999999999999289 ) ) ;
#1487=CARTESIAN_POINT ( 'NONE',  ( 66.99999999999997158, -5.000000000000000000, 44.49999999999999289 ) ) ;
#1488=ORIENTED_EDGE ( 'NONE', *, *, #2475, .T. ) ;
#1490=FACE_OUTER_BOUND ( 'NONE', #2954, .T. ) ;
#1493=DIRECTION ( 'NONE',  ( -0.000000000000000000, 1.000000000000000000, -0.000000000000000000 ) ) ;
#1496=DIRECTION ( 'NONE',  ( -1.000000000000000000, -0.000000000000000000, -0.000000000000000000 ) ) ;
#1499=ADVANCED_FACE ( 'NONE', ( #2862 ), #771, .T. ) ;
#1500=ORIENTED_EDGE ( 'NONE', *, *, #1764, .T. ) ;
#1504=CARTESIAN_POINT ( 'NONE',  ( -66.99999999999997158, -5.000000000000000000, -41.99999999999999289 ) ) ;
#1509=CARTESIAN_POINT ( 'NONE',  ( 75.00000000000000000, 50.00000000000000000, -50.00000000000000000 ) ) ;
#1510=EDGE_CURVE ( 'NONE', #1277, #3026, #758, .T. ) ;
#1513=CARTESIAN_POINT ( 'NONE',  ( -66.99999999999997158, 0.000000000000000000, -41.99999999999999289 ) ) ;
#1514=CARTESIAN_POINT ( 'NONE',  ( -74.99999999999998579, 0.000000000000000000, -50.00000000000000000 ) ) ;
#1515=AXIS2_PLACEMENT_3D ( 'NONE', #557, #1585, #3230 ) ;
#1519=AXIS2_PLACEMENT_3D ( 'NONE', #2919, #2709, #2204 ) ;
#1521=ORIENTED_EDGE ( 'NONE', *, *, #603, .T. ) ;
#1524=VECTOR ( 'NONE', #1220, 999.9999999999998863 ) ;
#1525=CIRCLE ( 'NONE', #1956, 7.500000000000000000 ) ;
#1529=EDGE_LOOP ( 'NONE', ( #1381, #2933, #142, #1174 ) ) ;
#1533=DIRECTION ( 'NONE',  ( -0.000000000000000000, 1.000000000000000000, -0.000000000000000000 ) ) ;
#1534=FACE_OUTER_BOUND ( 'NONE', #1814, .T. ) ;
#1535=EDGE_CURVE ( 'NONE', #468, #2976, #1198, .T. ) ;
#1536=DIRECTION ( 'NONE',  ( 0.000000000000000000, -1.000000000000000000, 0.000000000000000000 ) ) ;
#1538=VERTEX_POINT ( 'NONE', #495 ) ;
#1539=VERTEX_POINT ( 'NONE', #1821 ) ;
#1543=FACE_OUTER_BOUND ( 'NONE', #1674, .T. ) ;
#1551=EDGE_CURVE ( 'NONE', #719, #35, #523, .T. ) ;
#1554=VERTEX_POINT ( 'NONE', #1807 ) ;
#1555=DIRECTION ( 'NONE',  ( -0.000000000000000000, 1.000000000000000000, -0.000000000000000000 ) ) ;
#1556=EDGE_CURVE ( 'NONE', #1570, #1763, #158, .T. ) ;
#1558=EDGE_LOOP ( 'NONE', ( #1692, #264, #2437 ) ) ;
#1559=FACE_BOUND ( 'NONE', #2192, .T. ) ;
#1561=EDGE_LOOP ( 'NONE', ( #2255, #1811 ) ) ;
#1567=DIRECTION ( 'NONE',  ( 1.000000000000000000, 0.000000000000000000, 0.000000000000000000 ) ) ;
#1570=VERTEX_POINT ( 'NONE', #1282 ) ;
#1571=CIRCLE ( 'NONE', #3269, 2.000000000000001776 ) ;
#1576=CONICAL_SURFACE ( 'NONE', #2554, 2.000000000000001776, 1.029744258676657642 ) ;
#1580=CIRCLE ( 'NONE', #2544, 2.000000000000001776 ) ;
#1581=ADVANCED_FACE ( 'NONE', ( #2559 ), #1589, .F. ) ;
#1585=DIRECTION ( 'NONE',  ( -0.000000000000000000, 1.000000000000000000, -0.000000000000000000 ) ) ;
#1589=CYLINDRICAL_SURFACE ( 'NONE', #3048, 2.000000000000001776 ) ;
#1592=EDGE_LOOP ( 'NONE', ( #2893, #3324 ) ) ;
#1594=ORIENTED_EDGE ( 'NONE', *, *, #2514, .F. ) ;
#1599=DIRECTION ( 'NONE',  ( -0.000000000000000000, 1.000000000000000000, -0.000000000000000000 ) ) ;
#1601=DIRECTION ( 'NONE',  ( 0.000000000000000000, 0.5150380749100514910, 0.8571673007021138879 ) ) ;
#1605=VERTEX_POINT ( 'NONE', #19 ) ;
#1609=CARTESIAN_POINT ( 'NONE',  ( 44.99999999999999289, 45.00000000000000711, -10.00000000000000533 ) ) ;
#1611=ORIENTED_EDGE ( 'NONE', *, *, #2350, .T. ) ;
#1613=( NAMED_UNIT ( * ) PLANE_ANGLE_UNIT ( ) SI_UNIT ( $, .RADIAN. ) );
#1618=EDGE_LOOP ( 'NONE', ( #4, #2118, #226, #2844 ) ) ;
#1619=EDGE_LOOP ( 'NONE', ( #2362, #3177, #1371, #1140 ) ) ;
#1620=DIRECTION ( 'NONE',  ( 0.000000000000000000, 0.5150380749100514910, 0.8571673007021138879 ) ) ;
#1626=EDGE_CURVE ( 'NONE', #3026, #1277, #980, .T. ) ;
#1629=VECTOR ( 'NONE', #1567, 1000.000000000000000 ) ;
#1634=COLOUR_RGB ( '',0.8941176470588234615, 0.8941176470588234615, 0.8941176470588234615 ) ;
#1635=DIRECTION ( 'NONE',  ( 0.000000000000000000, 0.000000000000000000, 1.000000000000000000 ) ) ;
#1639=ORIENTED_EDGE ( 'NONE', *, *, #1535, .T. ) ;
#1640=ORIENTED_EDGE ( 'NONE', *, *, #248, .T. ) ;
#1642=FACE_BOUND ( 'NONE', #1265, .T. ) ;
#1643=DIRECTION ( 'NONE',  ( 1.387778780781445676E-16, 0.000000000000000000, -1.000000000000000000 ) ) ;
#1652=CARTESIAN_POINT ( 'NONE',  ( 45.00000000000000000, 50.00000000000000000, 9.999999999999994671 ) ) ;
#1653=CARTESIAN_POINT ( 'NONE',  ( 44.99999999999999289, 45.00000000000000711, -8.000000000000003553 ) ) ;
#1654=CARTESIAN_POINT ( 'NONE',  ( -45.00000000000000000, 45.00000000000000711, -11.99999999999999645 ) ) ;
#1667=EDGE_CURVE ( 'NONE', #824, #113, #82, .T. ) ;
#1668=DIRECTION ( 'NONE',  ( 1.000000000000000000, 0.000000000000000000, -0.000000000000000000 ) ) ;
#1669=VECTOR ( 'NONE', #2214, 1000.000000000000000 ) ;
#1674=EDGE_LOOP ( 'NONE', ( #2406, #735, #679, #238 ) ) ;
#1680=ADVANCED_FACE ( 'NONE', ( #1117 ), #50, .F. ) ;
#1683=DIRECTION ( 'NONE',  ( -0.000000000000000000, 1.000000000000000000, -0.000000000000000000 ) ) ;
#1691=AXIS2_PLACEMENT_3D ( 'NONE', #1246, #939, #3018 ) ;
#1692=ORIENTED_EDGE ( 'NONE', *, *, #310, .F. ) ;
#1694=LINE ( 'NONE', #956, #432 ) ;
#1703=CARTESIAN_POINT ( 'NONE',  ( -66.99999999999997158, 0.000000000000000000, 39.50000000000000000 ) ) ;
#1704=CARTESIAN_POINT ( 'NONE',  ( 66.99999999999997158, -5.000000000000000000, -41.99999999999999289 ) ) ;
#1707=DIRECTION ( 'NONE',  ( 1.000000000000000000, 0.000000000000000000, 0.000000000000000000 ) ) ;
#1718=DIRECTION ( 'NONE',  ( -0.000000000000000000, -0.000000000000000000, 1.000000000000000000 ) ) ;
#1720=DIRECTION ( 'NONE',  ( 0.000000000000000000, 0.000000000000000000, 1.000000000000000000 ) ) ;
#1724=EDGE_LOOP ( 'NONE', ( #208, #88 ) ) ;
#1726=EDGE_LOOP ( 'NONE', ( #203, #1025, #454, #2305 ) ) ;
#1727=EDGE_CURVE ( 'NONE', #1875, #1319, #1580, .T. ) ;
#1731=CONICAL_SURFACE ( 'NONE', #3157, 2.000000000000001776, 1.029744258676657642 ) ;
#1732=AXIS2_PLACEMENT_3D ( 'NONE', #1818, #2532, #2858 ) ;
#1739=PLANE ( 'NONE',  #1454 ) ;
#1741=VECTOR ( 'NONE', #148, 1000.000000000000000 ) ;
#1747=EDGE_CURVE ( 'NONE', #2320, #719, #1078, .T. ) ;
#1749=ORIENTED_EDGE ( 'NONE', *, *, #1411, .F. ) ;
#1750=CARTESIAN_POINT ( 'NONE',  ( 45.00000000000000000, 43.79827876194489278, 9.999999999999994671 ) ) ;
#1755=CARTESIAN_POINT ( 'NONE',  ( -7.500000000000000000, 25.00000000000000000, 50.00000000000000000 ) ) ;
#1763=VERTEX_POINT ( 'NONE', #1393 ) ;
#1764=EDGE_CURVE ( 'NONE', #774, #561, #2432, .T. ) ;
#1767=LINE ( 'NONE', #246, #1027 ) ;
#1772=DIRECTION ( 'NONE',  ( 0.000000000000000000, 0.000000000000000000, -1.000000000000000000 ) ) ;
#1773=DIRECTION ( 'NONE',  ( -0.000000000000000000, 1.000000000000000000, -0.000000000000000000 ) ) ;
#1774=EDGE_LOOP ( 'NONE', ( #2358, #2785, #709 ) ) ;
#1778=FACE_BOUND ( 'NONE', #651, .T. ) ;
#1779=EDGE_CURVE ( 'NONE', #2115, #347, #2984, .T. ) ;
#1781=ORIENTED_EDGE ( 'NONE', *, *, #630, .T. ) ;
#1786=DIRECTION ( 'NONE',  ( 0.000000000000000000, 0.000000000000000000, 1.000000000000000000 ) ) ;
#1800=DIRECTION ( 'NONE',  ( 0.000000000000000000, -0.000000000000000000, -1.000000000000000000 ) ) ;
#1801=ORIENTED_EDGE ( 'NONE', *, *, #1852, .F. ) ;
#1803=DIRECTION ( 'NONE',  ( -0.000000000000000000, 1.000000000000000000, -0.000000000000000000 ) ) ;
#1807=CARTESIAN_POINT ( 'NONE',  ( 66.99999999999997158, -5.000000000000000000, -39.50000000000000000 ) ) ;
#1811=ORIENTED_EDGE ( 'NONE', *, *, #1556, .F. ) ;
#1814=EDGE_LOOP ( 'NONE', ( #562, #1344, #2718 ) ) ;
#1818=CARTESIAN_POINT ( 'NONE',  ( 0.000000000000000000, 25.00000000000000000, 47.00000000000000000 ) ) ;
#1819=( NAMED_UNIT ( * ) PLANE_ANGLE_UNIT ( ) SI_UNIT ( $, .RADIAN. ) );
#1820=CARTESIAN_POINT ( 'NONE',  ( 66.99999999999997158, 0.000000000000000000, 39.50000000000000000 ) ) ;
#1821=CARTESIAN_POINT ( 'NONE',  ( 45.00000000000000000, 50.00000000000000000, 7.999999999999992895 ) ) ;
#1823=EDGE_LOOP ( 'NONE', ( #950, #2865 ) ) ;
#1824=ORIENTED_EDGE ( 'NONE', *, *, #2802, .F. ) ;
#1826=EDGE_LOOP ( 'NONE', ( #2421, #551, #1010, #1500 ) ) ;
#1827=CARTESIAN_POINT ( 'NONE',  ( -66.99999999999997158, -5.000000000000000000, 41.99999999999999289 ) ) ;
#1828=CLOSED_SHELL ( 'NONE', ( #3339, #93, #362, #1680, #1456, #3315, #118, #1004, #633, #2560, #2361, #3191, #2610, #2538, #2953, #2707, #400, #2387, #1233, #425, #2453, #2428, #76, #1921, #2286, #953, #992, #492, #1499, #2631, #2731, #1929, #2201, #2088, #1218, #1581, #2161 ) ) ;
#1832=DIRECTION ( 'NONE',  ( 0.000000000000000000, 0.000000000000000000, 1.000000000000000000 ) ) ;
#1836=DIRECTION ( 'NONE',  ( 0.000000000000000000, 0.000000000000000000, 1.000000000000000000 ) ) ;
#1841=VECTOR ( 'NONE', #3012, 1000.000000000000000 ) ;
#1852=EDGE_CURVE ( 'NONE', #121, #3215, #3330, .T. ) ;
#1853=AXIS2_PLACEMENT_3D ( 'NONE', #768, #2368, #2878 ) ;
#1864=PLANE ( 'NONE',  #811 ) ;
#1868=ORIENTED_EDGE ( 'NONE', *, *, #1288, .T. ) ;
#1869=EDGE_CURVE ( 'NONE', #531, #2478, #2777, .T. ) ;
#1871=CARTESIAN_POINT ( 'NONE',  ( 0.000000000000000000, 0.000000000000000000, 0.000000000000000000 ) ) ;
#1873=DIRECTION ( 'NONE',  ( 0.000000000000000000, 0.000000000000000000, 1.000000000000000000 ) ) ;
#1875=VERTEX_POINT ( 'NONE', #3016 ) ;
#1876=EDGE_CURVE ( 'NONE', #3215, #121, #1946, .T. ) ;
#1877=ORIENTED_EDGE ( 'NONE', *, *, #1160, .T. ) ;
#1880=EDGE_LOOP ( 'NONE', ( #763, #999 ) ) ;
#1881=DIRECTION ( 'NONE',  ( -1.387778780781445676E-16, -0.000000000000000000, 1.000000000000000000 ) ) ;
#1883=EDGE_LOOP ( 'NONE', ( #1982, #2294, #933, #2811 ) ) ;
#1884=DIRECTION ( 'NONE',  ( 1.000000000000000000, 0.000000000000000000, 0.000000000000000000 ) ) ;
#1898=AXIS2_PLACEMENT_3D ( 'NONE', #2730, #1137, #1421 ) ;
#1901=AXIS2_PLACEMENT_3D ( 'NONE', #119, #2689, #1668 ) ;
#1902=AXIS2_PLACEMENT_3D ( 'NONE', #3238, #58, #1106 ) ;
#1905=STYLED_ITEM ( 'NONE', ( #620 ), #479 ) ;
#1906=( LENGTH_UNIT ( ) NAMED_UNIT ( * ) SI_UNIT ( .MILLI., .METRE. ) );
#1907=LINE ( 'NONE', #2950, #2385 ) ;
#1909=DIRECTION ( 'NONE',  ( 0.000000000000000000, -1.000000000000000000, 0.000000000000000000 ) ) ;
#1911=ORIENTED_EDGE ( 'NONE', *, *, #2324, .T. ) ;
#1914=VECTOR ( 'NONE', #1139, 1000.000000000000000 ) ;
#1915=CARTESIAN_POINT ( 'NONE',  ( 66.99999999999997158, 0.000000000000000000, -41.99999999999999289 ) ) ;
#1921=ADVANCED_FACE ( 'NONE', ( #673 ), #661, .T. ) ;
#1922=PLANE ( 'NONE',  #532 ) ;
#1925=LINE ( 'NONE', #1654, #324 ) ;
#1927=ORIENTED_EDGE ( 'NONE', *, *, #1481, .F. ) ;
#1928=CARTESIAN_POINT ( 'NONE',  ( 45.00000000000000000, 50.00000000000000000, 7.999999999999992895 ) ) ;
#1929=ADVANCED_FACE ( 'NONE', ( #2261 ), #2737, .F. ) ;
#1932=CARTESIAN_POINT ( 'NONE',  ( 44.99999999999999289, 43.79827876194489278, -10.00000000000000533 ) ) ;
#1935=FACE_OUTER_BOUND ( 'NONE', #3201, .T. ) ;
#1936=CYLINDRICAL_SURFACE ( 'NONE', #3318, 7.500000000000000000 ) ;
#1937=DIRECTION ( 'NONE',  ( 0.000000000000000000, 0.000000000000000000, 1.000000000000000000 ) ) ;
#1939=LINE ( 'NONE', #170, #1669 ) ;
#1943=ORIENTED_EDGE ( 'NONE', *, *, #43, .T. ) ;
#1946=CIRCLE ( 'NONE', #1349, 2.499999999999995115 ) ;
#1947=CIRCLE ( 'NONE', #861, 2.000000000000001776 ) ;
#1954=MECHANICAL_DESIGN_GEOMETRIC_PRESENTATION_REPRESENTATION('',(#3274),#2771);
#1956=AXIS2_PLACEMENT_3D ( 'NONE', #2472, #368, #2457 ) ;
#1960=EDGE_CURVE ( 'NONE', #2478, #3154, #1525, .T. ) ;
#1964=CIRCLE ( 'NONE', #757, 2.000000000000001776 ) ;
#1968=VERTEX_POINT ( 'NONE', #1166 ) ;
#1970=EDGE_CURVE ( 'NONE', #113, #277, #2199, .T. ) ;
#1974=CYLINDRICAL_SURFACE ( 'NONE', #1691, 2.499999999999995115 ) ;
#1976=CARTESIAN_POINT ( 'NONE',  ( -44.99999999999999289, 50.00000000000000000, 10.00000000000000533 ) ) ;
#1982=ORIENTED_EDGE ( 'NONE', *, *, #2514, .T. ) ;
#1983=DIRECTION ( 'NONE',  ( 0.000000000000000000, 0.000000000000000000, 1.000000000000000000 ) ) ;
#1988=CARTESIAN_POINT ( 'NONE',  ( 66.99999999999997158, -5.000000000000000000, 39.50000000000000000 ) ) ;
#1991=EDGE_CURVE ( 'NONE', #824, #2761, #2790, .T. ) ;
#1995=CARTESIAN_POINT ( 'NONE',  ( -45.00000000000000000, 45.00000000000000711, -9.999999999999994671 ) ) ;
#1998=EDGE_CURVE ( 'NONE', #480, #1538, #728, .T. ) ;
#2001=AXIS2_PLACEMENT_3D ( 'NONE', #1114, #1391, #1832 ) ;
#2012=DIRECTION ( 'NONE',  ( 1.049727191138620668E-16, 0.5150380749100514910, -0.8571673007021138879 ) ) ;
#2019=DIRECTION ( 'NONE',  ( 0.000000000000000000, 0.000000000000000000, 1.000000000000000000 ) ) ;
#2024=FACE_OUTER_BOUND ( 'NONE', #2788, .T. ) ;
#2027=CYLINDRICAL_SURFACE ( 'NONE', #1732, 7.500000000000000000 ) ;
#2028=CARTESIAN_POINT ( 'NONE',  ( 44.99999999999999289, 50.00000000000000000, -8.000000000000003553 ) ) ;
#2030=APPLICATION_CONTEXT ( 'automotive_design' ) ;
#2032=DIRECTION ( 'NONE',  ( -0.000000000000000000, 1.000000000000000000, -0.000000000000000000 ) ) ;
#2035=ORIENTED_EDGE ( 'NONE', *, *, #1779, .T. ) ;
#2044=CARTESIAN_POINT ( 'NONE',  ( -66.99999999999997158, 0.000000000000000000, -39.50000000000000000 ) ) ;
#2056=CARTESIAN_POINT ( 'NONE',  ( -66.99999999999997158, -5.000000000000000000, -41.99999999999999289 ) ) ;
#2058=VECTOR ( 'NONE', #2627, 1000.000000000000000 ) ;
#2061=CIRCLE ( 'NONE', #584, 2.000000000000001776 ) ;
#2065=CARTESIAN_POINT ( 'NONE',  ( 66.99999999999997158, -5.000000000000000000, 41.99999999999999289 ) ) ;
#2074=AXIS2_PLACEMENT_3D ( 'NONE', #3285, #1773, #696 ) ;
#2075=CONICAL_SURFACE ( 'NONE', #1853, 2.000000000000001776, 1.029744258676657642 ) ;
#2077=DIRECTION ( 'NONE',  ( -0.000000000000000000, 1.000000000000000000, -0.000000000000000000 ) ) ;
#2084=DIRECTION ( 'NONE',  ( 0.000000000000000000, 0.000000000000000000, 1.000000000000000000 ) ) ;
#2086=VERTEX_POINT ( 'NONE', #2160 ) ;
#2088=ADVANCED_FACE ( 'NONE', ( #813 ), #1327, .F. ) ;
#2089=ORIENTED_EDGE ( 'NONE', *, *, #2696, .F. ) ;
#2090=DIRECTION ( 'NONE',  ( -0.000000000000000000, 1.000000000000000000, -0.000000000000000000 ) ) ;
#2095=FACE_OUTER_BOUND ( 'NONE', #982, .T. ) ;
#2098=CARTESIAN_POINT ( 'NONE',  ( 45.00000000000000000, 45.00000000000000711, 9.999999999999994671 ) ) ;
#2104=PLANE ( 'NONE',  #3043 ) ;
#2106=VERTEX_POINT ( 'NONE', #2874 ) ;
#2109=VECTOR ( 'NONE', #2847, 1000.000000000000000 ) ;
#2110=LINE ( 'NONE', #1130, #2873 ) ;
#2111=CARTESIAN_POINT ( 'NONE',  ( -75.00000000000000000, 50.00000000000000000, 50.00000000000000000 ) ) ;
#2115=VERTEX_POINT ( 'NONE', #1359 ) ;
#2116=AXIS2_PLACEMENT_3D ( 'NONE', #2998, #2483, #657 ) ;
#2118=ORIENTED_EDGE ( 'NONE', *, *, #1535, .F. ) ;
#2120=AXIS2_PLACEMENT_3D ( 'NONE', #2056, #2598, #504 ) ;
#2125=CIRCLE ( 'NONE', #2074, 2.000000000000001776 ) ;
#2127=CARTESIAN_POINT ( 'NONE',  ( -66.99999999999997158, -5.000000000000000000, 44.49999999999999289 ) ) ;
#2128=( GEOMETRIC_REPRESENTATION_CONTEXT ( 3 ) GLOBAL_UNCERTAINTY_ASSIGNED_CONTEXT ( ( #553 ) ) GLOBAL_UNIT_ASSIGNED_CONTEXT ( ( #1906, #1613, #2414 ) ) REPRESENTATION_CONTEXT ( 'NONE', 'WORKASPACE' ) );
#2132=EDGE_CURVE ( 'NONE', #3190, #531, #917, .T. ) ;
#2136=DIRECTION ( 'NONE',  ( 0.000000000000000000, 0.5150380749100514910, 0.8571673007021138879 ) ) ;
#2144=DIRECTION ( 'NONE',  ( 0.000000000000000000, 0.000000000000000000, 1.000000000000000000 ) ) ;
#2152=ORIENTED_EDGE ( 'NONE', *, *, #777, .F. ) ;
#2155=ORIENTED_EDGE ( 'NONE', *, *, #646, .F. ) ;
#2160=CARTESIAN_POINT ( 'NONE',  ( -44.99999999999999289, 43.79827876194489278, 10.00000000000000533 ) ) ;
#2161=ADVANCED_FACE ( 'NONE', ( #2400 ), #1731, .F. ) ;
#2166=ORIENTED_EDGE ( 'NONE', *, *, #2576, .T. ) ;
#2170=CARTESIAN_POINT ( 'NONE',  ( 44.99999999999999289, 45.00000000000000711, -10.00000000000000533 ) ) ;
#2173=VECTOR ( 'NONE', #893, 1000.000000000000000 ) ;
#2176=AXIS2_PLACEMENT_3D ( 'NONE', #2170, #3222, #875 ) ;
#2183=VECTOR ( 'NONE', #3297, 1000.000000000000000 ) ;
#2185=DIRECTION ( 'NONE',  ( -0.000000000000000000, -1.000000000000000000, -0.000000000000000000 ) ) ;
#2187=CARTESIAN_POINT ( 'NONE',  ( -66.99999999999997158, -5.000000000000000000, -39.50000000000000000 ) ) ;
#2192=EDGE_LOOP ( 'NONE', ( #2885, #1417 ) ) ;
#2198=CARTESIAN_POINT ( 'NONE',  ( -66.99999999999997158, -5.000000000000000000, -44.49999999999999289 ) ) ;
#2199=LINE ( 'NONE', #2028, #3095 ) ;
#2201=ADVANCED_FACE ( 'NONE', ( #3204 ), #3039, .F. ) ;
#2202=EDGE_LOOP ( 'NONE', ( #812, #2681, #3113, #1321 ) ) ;
#2204=DIRECTION ( 'NONE',  ( 0.000000000000000000, 0.000000000000000000, 1.000000000000000000 ) ) ;
#2205=EDGE_CURVE ( 'NONE', #2259, #277, #1571, .T. ) ;
#2206=ORIENTED_EDGE ( 'NONE', *, *, #2257, .T. ) ;
#2209=ORIENTED_EDGE ( 'NONE', *, *, #325, .F. ) ;
#2211=EDGE_CURVE ( 'NONE', #2585, #35, #2625, .T. ) ;
#2212=CARTESIAN_POINT ( 'NONE',  ( 75.00000000000000000, 50.00000000000000000, -50.00000000000000000 ) ) ;
#2214=DIRECTION ( 'NONE',  ( 1.000000000000000000, 0.000000000000000000, 0.000000000000000000 ) ) ;
#2219=EDGE_CURVE ( 'NONE', #1968, #2106, #3322, .T. ) ;
#2226=CIRCLE ( 'NONE', #1519, 2.000000000000001776 ) ;
#2227=AXIS2_PLACEMENT_3D ( 'NONE', #798, #252, #3372 ) ;
#2230=DIRECTION ( 'NONE',  ( 0.000000000000000000, 0.000000000000000000, 1.000000000000000000 ) ) ;
#2236=CARTESIAN_POINT ( 'NONE',  ( -44.99999999999999289, 45.00000000000000711, 8.000000000000003553 ) ) ;
#2248=CARTESIAN_POINT ( 'NONE',  ( 75.00000000000000000, 0.000000000000000000, 50.00000000000000000 ) ) ;
#2253=DIRECTION ( 'NONE',  ( -0.000000000000000000, 1.000000000000000000, -0.000000000000000000 ) ) ;
#2255=ORIENTED_EDGE ( 'NONE', *, *, #1149, .F. ) ;
#2257=EDGE_CURVE ( 'NONE', #2106, #1319, #1453, .T. ) ;
#2259=VERTEX_POINT ( 'NONE', #178 ) ;
#2261=FACE_OUTER_BOUND ( 'NONE', #1618, .T. ) ;
#2262=EDGE_CURVE ( 'NONE', #531, #3190, #2930, .T. ) ;
#2264=CARTESIAN_POINT ( 'NONE',  ( 45.00000000000000000, 50.00000000000000000, 9.999999999999994671 ) ) ;
#2268=ORIENTED_EDGE ( 'NONE', *, *, #891, .F. ) ;
#2269=CYLINDRICAL_SURFACE ( 'NONE', #206, 2.499999999999995115 ) ;
#2277=VECTOR ( 'NONE', #1881, 1000.000000000000000 ) ;
#2278=ORIENTED_EDGE ( 'NONE', *, *, #1250, .F. ) ;
#2280=CIRCLE ( 'NONE', #427, 2.000000000000001776 ) ;
#2282=LINE ( 'NONE', #1216, #2183 ) ;
#2286=ADVANCED_FACE ( 'NONE', ( #1935 ), #1922, .T. ) ;
#2287=DIRECTION ( 'NONE',  ( 0.000000000000000000, 0.000000000000000000, -1.000000000000000000 ) ) ;
#2290=ORIENTED_EDGE ( 'NONE', *, *, #3213, .F. ) ;
#2291=VERTEX_POINT ( 'NONE', #1439 ) ;
#2294=ORIENTED_EDGE ( 'NONE', *, *, #1998, .F. ) ;
#2302=DIRECTION ( 'NONE',  ( 0.000000000000000000, -1.000000000000000000, 0.000000000000000000 ) ) ;
#2305=ORIENTED_EDGE ( 'NONE', *, *, #1960, .T. ) ;
#2315=CARTESIAN_POINT ( 'NONE',  ( -66.99999999999997158, -5.000000000000000000, -39.50000000000000000 ) ) ;
#2320=VERTEX_POINT ( 'NONE', #1408 ) ;
#2324=EDGE_CURVE ( 'NONE', #1554, #1763, #2451, .T. ) ;
#2327=EDGE_LOOP ( 'NONE', ( #2734, #1801 ) ) ;
#2331=AXIS2_PLACEMENT_3D ( 'NONE', #2431, #81, #2402 ) ;
#2335=DIRECTION ( 'NONE',  ( 0.000000000000000000, 0.000000000000000000, 1.000000000000000000 ) ) ;
#2339=VECTOR ( 'NONE', #2656, 1000.000000000000000 ) ;
#2341=EDGE_LOOP ( 'NONE', ( #2524, #1153, #2035 ) ) ;
#2346=DIRECTION ( 'NONE',  ( -0.000000000000000000, 1.000000000000000000, -0.000000000000000000 ) ) ;
#2350=EDGE_CURVE ( 'NONE', #2691, #594, #382, .T. ) ;
#2351=DIRECTION ( 'NONE',  ( 0.000000000000000000, 0.000000000000000000, -1.000000000000000000 ) ) ;
#2355=CARTESIAN_POINT ( 'NONE',  ( -7.500000000000000000, 25.00000000000000000, 47.00000000000000000 ) ) ;
#2358=ORIENTED_EDGE ( 'NONE', *, *, #3058, .F. ) ;
#2360=CARTESIAN_POINT ( 'NONE',  ( 44.99999999999999289, 50.00000000000000000, -10.00000000000000533 ) ) ;
#2361=ADVANCED_FACE ( 'NONE', ( #1188 ), #1177, .T. ) ;
#2362=ORIENTED_EDGE ( 'NONE', *, *, #433, .F. ) ;
#2367=DIRECTION ( 'NONE',  ( -0.000000000000000000, -1.000000000000000000, -0.000000000000000000 ) ) ;
#2368=DIRECTION ( 'NONE',  ( -0.000000000000000000, 1.000000000000000000, -0.000000000000000000 ) ) ;
#2369=PLANE ( 'NONE',  #2331 ) ;
#2380=ORIENTED_EDGE ( 'NONE', *, *, #842, .F. ) ;
#2385=VECTOR ( 'NONE', #350, 1000.000000000000000 ) ;
#2387=ADVANCED_FACE ( 'NONE', ( #2545, #984, #1778, #1559, #2024 ), #466, .F. ) ;
#2391=DIRECTION ( 'NONE',  ( 0.000000000000000000, -1.000000000000000000, 0.000000000000000000 ) ) ;
#2392=VECTOR ( 'NONE', #39, 1000.000000000000000 ) ;
#2396=DIRECTION ( 'NONE',  ( 0.000000000000000000, 0.000000000000000000, 1.000000000000000000 ) ) ;
#2398=VERTEX_POINT ( 'NONE', #1750 ) ;
#2400=FACE_OUTER_BOUND ( 'NONE', #1774, .T. ) ;
#2402=DIRECTION ( 'NONE',  ( -1.000000000000000000, 0.000000000000000000, -0.000000000000000000 ) ) ;
#2406=ORIENTED_EDGE ( 'NONE', *, *, #603, .F. ) ;
#2410=CARTESIAN_POINT ( 'NONE',  ( 66.99999999999997158, -5.000000000000000000, -44.49999999999999289 ) ) ;
#2411=EDGE_CURVE ( 'NONE', #2972, #448, #209, .T. ) ;
#2413=CARTESIAN_POINT ( 'NONE',  ( -45.00000000000000000, 45.00000000000000711, -9.999999999999994671 ) ) ;
#2414=( NAMED_UNIT ( * ) SI_UNIT ( $, .STERADIAN. ) SOLID_ANGLE_UNIT ( ) );
#2415=CARTESIAN_POINT ( 'NONE',  ( -66.99999999999997158, -5.000000000000000000, 41.99999999999999289 ) ) ;
#2419=ORIENTED_EDGE ( 'NONE', *, *, #970, .T. ) ;
#2421=ORIENTED_EDGE ( 'NONE', *, *, #815, .T. ) ;
#2423=FACE_OUTER_BOUND ( 'NONE', #2936, .T. ) ;
#2428=ADVANCED_FACE ( 'NONE', ( #1543 ), #2786, .T. ) ;
#2430=( NAMED_UNIT ( * ) SI_UNIT ( $, .STERADIAN. ) SOLID_ANGLE_UNIT ( ) );
#2431=CARTESIAN_POINT ( 'NONE',  ( -75.00000000000000000, 50.00000000000000000, 50.00000000000000000 ) ) ;
#2432=LINE ( 'NONE', #96, #2717 ) ;
#2437=ORIENTED_EDGE ( 'NONE', *, *, #2696, .T. ) ;
#2438=VECTOR ( 'NONE', #1379, 1000.000000000000000 ) ;
#2439=FACE_OUTER_BOUND ( 'NONE', #2902, .T. ) ;
#2443=VECTOR ( 'NONE', #2492, 1000.000000000000000 ) ;
#2446=AXIS2_PLACEMENT_3D ( 'NONE', #2819, #3360, #3046 ) ;
#2451=LINE ( 'NONE', #115, #1841 ) ;
#2453=ADVANCED_FACE ( 'NONE', ( #1490 ), #453, .T. ) ;
#2457=DIRECTION ( 'NONE',  ( 1.000000000000000000, 0.000000000000000000, 0.000000000000000000 ) ) ;
#2460=VERTEX_POINT ( 'NONE', #191 ) ;
#2472=CARTESIAN_POINT ( 'NONE',  ( 0.000000000000000000, 25.00000000000000000, 50.00000000000000000 ) ) ;
#2475=EDGE_CURVE ( 'NONE', #3078, #499, #1300, .T. ) ;
#2476=CARTESIAN_POINT ( 'NONE',  ( -45.00000000000000000, 50.00000000000000000, -11.99999999999999645 ) ) ;
#2477=CARTESIAN_POINT ( 'NONE',  ( 45.00000000000000000, 45.00000000000000711, 9.999999999999994671 ) ) ;
#2478=VERTEX_POINT ( 'NONE', #227 ) ;
#2481=ORIENTED_EDGE ( 'NONE', *, *, #891, .T. ) ;
#2483=DIRECTION ( 'NONE',  ( -0.000000000000000000, 1.000000000000000000, -0.000000000000000000 ) ) ;
#2484=CARTESIAN_POINT ( 'NONE',  ( 7.500000000000000000, 25.00000000000000000, 47.00000000000000000 ) ) ;
#2485=CARTESIAN_POINT ( 'NONE',  ( 7.500000000000000000, 25.00000000000000000, 47.00000000000000000 ) ) ;
#2490=AXIS2_PLACEMENT_3D ( 'NONE', #421, #645, #1720 ) ;
#2492=DIRECTION ( 'NONE',  ( -0.000000000000000000, 1.000000000000000000, -0.000000000000000000 ) ) ;
#2500=AXIS2_PLACEMENT_3D ( 'NONE', #2940, #598, #1643 ) ;
#2514=EDGE_CURVE ( 'NONE', #35, #1538, #1324, .T. ) ;
#2520=DIRECTION ( 'NONE',  ( 0.000000000000000000, 0.000000000000000000, 1.000000000000000000 ) ) ;
#2523=LINE ( 'NONE', #2236, #1524 ) ;
#2524=ORIENTED_EDGE ( 'NONE', *, *, #611, .F. ) ;
#2531=ORIENTED_EDGE ( 'NONE', *, *, #310, .T. ) ;
#2532=DIRECTION ( 'NONE',  ( -0.000000000000000000, -0.000000000000000000, 1.000000000000000000 ) ) ;
#2535=LINE ( 'NONE', #2355, #2109 ) ;
#2538=ADVANCED_FACE ( 'NONE', ( #3151 ), #2104, .F. ) ;
#2544=AXIS2_PLACEMENT_3D ( 'NONE', #848, #1100, #590 ) ;
#2545=FACE_BOUND ( 'NONE', #1592, .T. ) ;
#2546=VECTOR ( 'NONE', #1493, 1000.000000000000000 ) ;
#2548=AXIS2_PLACEMENT_3D ( 'NONE', #1995, #3342, #1205 ) ;
#2553=AXIS2_PLACEMENT_3D ( 'NONE', #1504, #2077, #1275 ) ;
#2554=AXIS2_PLACEMENT_3D ( 'NONE', #597, #626, #2956 ) ;
#2557=AXIS2_PLACEMENT_3D ( 'NONE', #3210, #1909, #2653 ) ;
#2558=CARTESIAN_POINT ( 'NONE',  ( 44.99999999999999289, 50.00000000000000000, -8.000000000000003553 ) ) ;
#2559=FACE_OUTER_BOUND ( 'NONE', #2202, .T. ) ;
#2560=ADVANCED_FACE ( 'NONE', ( #11 ), #298, .T. ) ;
#2574=CARTESIAN_POINT ( 'NONE',  ( -75.00000000000000000, 0.000000000000000000, 50.00000000000000000 ) ) ;
#2576=EDGE_CURVE ( 'NONE', #2115, #801, #792, .T. ) ;
#2578=ORIENTED_EDGE ( 'NONE', *, *, #1876, .T. ) ;
#2585=VERTEX_POINT ( 'NONE', #1055 ) ;
#2586=CARTESIAN_POINT ( 'NONE',  ( -66.99999999999997158, -5.000000000000000000, -44.49999999999999289 ) ) ;
#2587=DIRECTION ( 'NONE',  ( -0.000000000000000000, 1.000000000000000000, -0.000000000000000000 ) ) ;
#2591=EDGE_LOOP ( 'NONE', ( #1640, #498, #1749, #345 ) ) ;
#2594=AXIS2_PLACEMENT_3D ( 'NONE', #2264, #1199, #2520 ) ;
#2595=EDGE_CURVE ( 'NONE', #113, #2761, #1964, .T. ) ;
#2598=DIRECTION ( 'NONE',  ( 0.000000000000000000, -1.000000000000000000, 0.000000000000000000 ) ) ;
#2599=EDGE_CURVE ( 'NONE', #3174, #3078, #3189, .T. ) ;
#2600=ORIENTED_EDGE ( 'NONE', *, *, #1852, .T. ) ;
#2605=DIRECTION ( 'NONE',  ( 0.000000000000000000, -1.000000000000000000, 0.000000000000000000 ) ) ;
#2609=VECTOR ( 'NONE', #1398, 1000.000000000000000 ) ;
#2610=ADVANCED_FACE ( 'NONE', ( #2905 ), #826, .T. ) ;
#2613=AXIS2_PLACEMENT_3D ( 'NONE', #1343, #2915, #2675 ) ;
#2617=AXIS2_PLACEMENT_3D ( 'NONE', #132, #420, #1462 ) ;
#2620=CARTESIAN_POINT ( 'NONE',  ( 75.00000000000000000, 50.00000000000000000, 50.00000000000000000 ) ) ;
#2625=LINE ( 'NONE', #286, #369 ) ;
#2627=DIRECTION ( 'NONE',  ( 0.000000000000000000, 0.000000000000000000, -1.000000000000000000 ) ) ;
#2631=ADVANCED_FACE ( 'NONE', ( #123 ), #330, .F. ) ;
#2633=DIRECTION ( 'NONE',  ( 0.000000000000000000, 0.000000000000000000, 1.000000000000000000 ) ) ;
#2636=EDGE_LOOP ( 'NONE', ( #3131, #1113 ) ) ;
#2637=DIRECTION ( 'NONE',  ( 0.000000000000000000, 0.000000000000000000, 1.000000000000000000 ) ) ;
#2639=DIRECTION ( 'NONE',  ( 1.000000000000000000, 0.000000000000000000, 0.000000000000000000 ) ) ;
#2652=EDGE_CURVE ( 'NONE', #1319, #1875, #2226, .T. ) ;
#2653=DIRECTION ( 'NONE',  ( 0.000000000000000000, 0.000000000000000000, 1.000000000000000000 ) ) ;
#2656=DIRECTION ( 'NONE',  ( -1.387778780781445676E-16, -0.000000000000000000, 1.000000000000000000 ) ) ;
#2663=AXIS2_PLACEMENT_3D ( 'NONE', #3080, #737, #1800 ) ;
#2664=AXIS2_PLACEMENT_3D ( 'NONE', #2065, #2302, #2084 ) ;
#2665=CARTESIAN_POINT ( 'NONE',  ( -66.99999999999997158, 0.000000000000000000, -44.49999999999999289 ) ) ;
#2673=DIRECTION ( 'NONE',  ( -0.000000000000000000, 1.000000000000000000, -0.000000000000000000 ) ) ;
#2675=DIRECTION ( 'NONE',  ( 0.000000000000000000, 0.000000000000000000, -1.000000000000000000 ) ) ;
#2677=ORIENTED_EDGE ( 'NONE', *, *, #2576, .F. ) ;
#2678=CARTESIAN_POINT ( 'NONE',  ( 0.000000000000000000, 0.000000000000000000, 0.000000000000000000 ) ) ;
#2681=ORIENTED_EDGE ( 'NONE', *, *, #2219, .F. ) ;
#2682=CARTESIAN_POINT ( 'NONE',  ( -75.00000000000000000, 0.000000000000000000, 50.00000000000000000 ) ) ;
#2687=DIRECTION ( 'NONE',  ( 0.000000000000000000, 0.000000000000000000, 1.000000000000000000 ) ) ;
#2689=DIRECTION ( 'NONE',  ( 0.000000000000000000, 0.000000000000000000, 1.000000000000000000 ) ) ;
#2691=VERTEX_POINT ( 'NONE', #2665 ) ;
#2696=EDGE_CURVE ( 'NONE', #2976, #468, #2280, .T. ) ;
#2704=EDGE_LOOP ( 'NONE', ( #429, #2531, #1639 ) ) ;
#2706=AXIS2_PLACEMENT_3D ( 'NONE', #2951, #832, #1873 ) ;
#2707=ADVANCED_FACE ( 'NONE', ( #837 ), #3200, .F. ) ;
#2709=DIRECTION ( 'NONE',  ( -0.000000000000000000, 1.000000000000000000, -0.000000000000000000 ) ) ;
#2712=CARTESIAN_POINT ( 'NONE',  ( -74.99999999999998579, 50.00000000000000000, -50.00000000000000000 ) ) ;
#2717=VECTOR ( 'NONE', #2185, 1000.000000000000000 ) ;
#2718=ORIENTED_EDGE ( 'NONE', *, *, #646, .T. ) ;
#2724=DIRECTION ( 'NONE',  ( -0.000000000000000000, 1.000000000000000000, -0.000000000000000000 ) ) ;
#2727=LINE ( 'NONE', #407, #1741 ) ;
#2730=CARTESIAN_POINT ( 'NONE',  ( 44.99999999999999289, 50.00000000000000000, -10.00000000000000533 ) ) ;
#2731=ADVANCED_FACE ( 'NONE', ( #2423 ), #3216, .F. ) ;
#2734=ORIENTED_EDGE ( 'NONE', *, *, #1876, .F. ) ;
#2737=CYLINDRICAL_SURFACE ( 'NONE', #1190, 2.000000000000001776 ) ;
#2745=FACE_OUTER_BOUND ( 'NONE', #1152, .T. ) ;
#2752=CARTESIAN_POINT ( 'NONE',  ( 45.00000000000000000, 50.00000000000000000, 9.999999999999994671 ) ) ;
#2754=CARTESIAN_POINT ( 'NONE',  ( 45.00000000000000000, 50.00000000000000000, 11.99999999999999645 ) ) ;
#2756=ORIENTED_EDGE ( 'NONE', *, *, #3206, .T. ) ;
#2761=VERTEX_POINT ( 'NONE', #1183 ) ;
#2769=CIRCLE ( 'NONE', #695, 2.499999999999995115 ) ;
#2770=DIRECTION ( 'NONE',  ( 0.000000000000000000, 0.000000000000000000, 1.000000000000000000 ) ) ;
#2771=( GEOMETRIC_REPRESENTATION_CONTEXT ( 3 ) GLOBAL_UNCERTAINTY_ASSIGNED_CONTEXT ( ( #77 ) ) GLOBAL_UNIT_ASSIGNED_CONTEXT ( ( #1447, #678, #426 ) ) REPRESENTATION_CONTEXT ( 'NONE', 'WORKASPACE' ) );
#2772=AXIS2_PLACEMENT_3D ( 'NONE', #234, #3351, #2287 ) ;
#2777=LINE ( 'NONE', #2485, #213 ) ;
#2784=EDGE_CURVE ( 'NONE', #895, #3174, #1252, .T. ) ;
#2785=ORIENTED_EDGE ( 'NONE', *, *, #1250, .T. ) ;
#2786=CYLINDRICAL_SURFACE ( 'NONE', #2553, 2.499999999999995115 ) ;
#2788=EDGE_LOOP ( 'NONE', ( #748, #2996, #1104, #1943 ) ) ;
#2790=LINE ( 'NONE', #656, #1403 ) ;
#2792=MANIFOLD_SOLID_BREP ( 'AdvancedHole1', #1828 ) ;
#2799=EDGE_LOOP ( 'NONE', ( #835, #3332, #376, #564 ) ) ;
#2801=ORIENTED_EDGE ( 'NONE', *, *, #325, .T. ) ;
#2802=EDGE_CURVE ( 'NONE', #2086, #2115, #2523, .T. ) ;
#2806=EDGE_CURVE ( 'NONE', #347, #2115, #2125, .T. ) ;
#2811=ORIENTED_EDGE ( 'NONE', *, *, #2211, .T. ) ;
#2816=SHAPE_DEFINITION_REPRESENTATION ( #1459, #685 ) ;
#2817=ORIENTED_EDGE ( 'NONE', *, *, #1626, .F. ) ;
#2818=VECTOR ( 'NONE', #2136, 999.9999999999998863 ) ;
#2819=CARTESIAN_POINT ( 'NONE',  ( -66.99999999999997158, 0.000000000000000000, 41.99999999999999289 ) ) ;
#2831=DIRECTION ( 'NONE',  ( -0.000000000000000000, 1.000000000000000000, -0.000000000000000000 ) ) ;
#2844=ORIENTED_EDGE ( 'NONE', *, *, #32, .T. ) ;
#2846=DIRECTION ( 'NONE',  ( 0.000000000000000000, 0.000000000000000000, 1.000000000000000000 ) ) ;
#2847=DIRECTION ( 'NONE',  ( -0.000000000000000000, -0.000000000000000000, 1.000000000000000000 ) ) ;
#2858=DIRECTION ( 'NONE',  ( 1.000000000000000000, 0.000000000000000000, 0.000000000000000000 ) ) ;
#2862=FACE_OUTER_BOUND ( 'NONE', #2871, .T. ) ;
#2865=ORIENTED_EDGE ( 'NONE', *, *, #1288, .F. ) ;
#2871=EDGE_LOOP ( 'NONE', ( #888, #2908 ) ) ;
#2873=VECTOR ( 'NONE', #1601, 999.9999999999998863 ) ;
#2874=CARTESIAN_POINT ( 'NONE',  ( -45.00000000000000000, 45.00000000000000711, -11.99999999999999645 ) ) ;
#2878=DIRECTION ( 'NONE',  ( 0.000000000000000000, 0.000000000000000000, 1.000000000000000000 ) ) ;
#2879=DIRECTION ( 'NONE',  ( -0.000000000000000000, 1.000000000000000000, -0.000000000000000000 ) ) ;
#2885=ORIENTED_EDGE ( 'NONE', *, *, #443, .F. ) ;
#2893=ORIENTED_EDGE ( 'NONE', *, *, #1727, .F. ) ;
#2897=CARTESIAN_POINT ( 'NONE',  ( -44.99999999999999289, 45.00000000000000711, 10.00000000000000533 ) ) ;
#2902=EDGE_LOOP ( 'NONE', ( #1824, #1135, #411 ) ) ;
#2903=DIRECTION ( 'NONE',  ( 0.000000000000000000, -1.000000000000000000, 0.000000000000000000 ) ) ;
#2904=EDGE_LOOP ( 'NONE', ( #1326, #2206, #41, #292 ) ) ;
#2905=FACE_OUTER_BOUND ( 'NONE', #3286, .T. ) ;
#2908=ORIENTED_EDGE ( 'NONE', *, *, #2132, .T. ) ;
#2910=CARTESIAN_POINT ( 'NONE',  ( -45.00000000000000000, 45.00000000000000711, -9.999999999999994671 ) ) ;
#2912=FILL_AREA_STYLE_COLOUR ( '', #1634 ) ;
#2915=DIRECTION ( 'NONE',  ( 0.000000000000000000, -1.000000000000000000, 0.000000000000000000 ) ) ;
#2919=CARTESIAN_POINT ( 'NONE',  ( -45.00000000000000000, 50.00000000000000000, -9.999999999999994671 ) ) ;
#2926=DIRECTION ( 'NONE',  ( 0.000000000000000000, 0.000000000000000000, 1.000000000000000000 ) ) ;
#2930=CIRCLE ( 'NONE', #97, 7.500000000000000000 ) ;
#2932=CARTESIAN_POINT ( 'NONE',  ( 66.99999999999997158, -5.000000000000000000, 39.50000000000000000 ) ) ;
#2933=ORIENTED_EDGE ( 'NONE', *, *, #2211, .F. ) ;
#2936=EDGE_LOOP ( 'NONE', ( #461, #2941, #26 ) ) ;
#2939=VECTOR ( 'NONE', #1620, 999.9999999999998863 ) ;
#2940=CARTESIAN_POINT ( 'NONE',  ( -75.00000000000000000, 50.00000000000000000, 50.00000000000000000 ) ) ;
#2941=ORIENTED_EDGE ( 'NONE', *, *, #1667, .T. ) ;
#2942=LINE ( 'NONE', #1425, #2173 ) ;
#2946=ORIENTED_EDGE ( 'NONE', *, *, #511, .T. ) ;
#2950=CARTESIAN_POINT ( 'NONE',  ( 44.99999999999999289, 50.00000000000000000, -12.00000000000000711 ) ) ;
#2951=CARTESIAN_POINT ( 'NONE',  ( -44.99999999999999289, 50.00000000000000000, 10.00000000000000533 ) ) ;
#2952=CARTESIAN_POINT ( 'NONE',  ( -66.99999999999997158, 0.000000000000000000, 44.49999999999999289 ) ) ;
#2953=ADVANCED_FACE ( 'NONE', ( #623 ), #1333, .F. ) ;
#2954=EDGE_LOOP ( 'NONE', ( #1133, #1184 ) ) ;
#2955=ORIENTED_EDGE ( 'NONE', *, *, #2599, .F. ) ;
#2956=DIRECTION ( 'NONE',  ( 0.000000000000000000, 0.000000000000000000, 1.000000000000000000 ) ) ;
#2962=DIRECTION ( 'NONE',  ( 0.000000000000000000, -1.000000000000000000, 0.000000000000000000 ) ) ;
#2969=ORIENTED_EDGE ( 'NONE', *, *, #1304, .T. ) ;
#2972=VERTEX_POINT ( 'NONE', #2187 ) ;
#2976=VERTEX_POINT ( 'NONE', #323 ) ;
#2983=CARTESIAN_POINT ( 'NONE',  ( -66.99999999999997158, -5.000000000000000000, -41.99999999999999289 ) ) ;
#2984=CIRCLE ( 'NONE', #1257, 2.000000000000001776 ) ;
#2991=DIRECTION ( 'NONE',  ( 0.000000000000000000, -1.000000000000000000, 0.000000000000000000 ) ) ;
#2992=AXIS2_PLACEMENT_3D ( 'NONE', #731, #1536, #1772 ) ;
#2996=ORIENTED_EDGE ( 'NONE', *, *, #1411, .T. ) ;
#2997=EDGE_CURVE ( 'NONE', #774, #2320, #1119, .T. ) ;
#2998=CARTESIAN_POINT ( 'NONE',  ( 66.99999999999997158, -5.000000000000000000, -41.99999999999999289 ) ) ;
#3005=FACE_OUTER_BOUND ( 'NONE', #2904, .T. ) ;
#3006=DIRECTION ( 'NONE',  ( 0.000000000000000000, 0.000000000000000000, 1.000000000000000000 ) ) ;
#3008=ORIENTED_EDGE ( 'NONE', *, *, #2806, .F. ) ;
#3012=DIRECTION ( 'NONE',  ( -0.000000000000000000, 1.000000000000000000, -0.000000000000000000 ) ) ;
#3016=CARTESIAN_POINT ( 'NONE',  ( -45.00000000000000000, 50.00000000000000000, -7.999999999999992895 ) ) ;
#3018=DIRECTION ( 'NONE',  ( 0.000000000000000000, 0.000000000000000000, 1.000000000000000000 ) ) ;
#3026=VERTEX_POINT ( 'NONE', #2932 ) ;
#3034=DIRECTION ( 'NONE',  ( -0.000000000000000000, 1.000000000000000000, -0.000000000000000000 ) ) ;
#3036=CIRCLE ( 'NONE', #913, 2.000000000000001776 ) ;
#3038=CARTESIAN_POINT ( 'NONE',  ( 66.99999999999997158, -5.000000000000000000, 41.99999999999999289 ) ) ;
#3039=CONICAL_SURFACE ( 'NONE', #1515, 2.000000000000001776, 1.029744258676657642 ) ;
#3043=AXIS2_PLACEMENT_3D ( 'NONE', #2620, #282, #2396 ) ;
#3045=AXIS2_PLACEMENT_3D ( 'NONE', #1976, #3034, #3251 ) ;
#3046=DIRECTION ( 'NONE',  ( 0.000000000000000000, 0.000000000000000000, -1.000000000000000000 ) ) ;
#3048=AXIS2_PLACEMENT_3D ( 'NONE', #473, #2831, #1007 ) ;
#3052=DIRECTION ( 'NONE',  ( 0.000000000000000000, -1.000000000000000000, 0.000000000000000000 ) ) ;
#3058=EDGE_CURVE ( 'NONE', #2460, #2106, #1925, .T. ) ;
#3066=CARTESIAN_POINT ( 'NONE',  ( 0.000000000000000000, 50.00000000000000000, 0.000000000000000000 ) ) ;
#3072=DIRECTION ( 'NONE',  ( -0.000000000000000000, 1.000000000000000000, -0.000000000000000000 ) ) ;
#3078=VERTEX_POINT ( 'NONE', #2952 ) ;
#3079=EDGE_CURVE ( 'NONE', #1554, #1605, #1201, .T. ) ;
#3080=CARTESIAN_POINT ( 'NONE',  ( -66.99999999999997158, -5.000000000000000000, 41.99999999999999289 ) ) ;
#3082=ORIENTED_EDGE ( 'NONE', *, *, #2784, .F. ) ;
#3095=VECTOR ( 'NONE', #2587, 1000.000000000000000 ) ;
#3105=AXIS2_PLACEMENT_3D ( 'NONE', #1827, #1352, #1173 ) ;
#3106=AXIS2_PLACEMENT_3D ( 'NONE', #1296, #2032, #1836 ) ;
#3107=DIRECTION ( 'NONE',  ( 0.000000000000000000, 0.000000000000000000, 1.000000000000000000 ) ) ;
#3111=AXIS2_PLACEMENT_3D ( 'NONE', #1871, #3207, #2639 ) ;
#3113=ORIENTED_EDGE ( 'NONE', *, *, #3182, .T. ) ;
#3127=CARTESIAN_POINT ( 'NONE',  ( 44.99999999999999289, 45.00000000000000711, -10.00000000000000533 ) ) ;
#3131=ORIENTED_EDGE ( 'NONE', *, *, #3134, .F. ) ;
#3132=FACE_OUTER_BOUND ( 'NONE', #3359, .T. ) ;
#3134=EDGE_CURVE ( 'NONE', #594, #2691, #1151, .T. ) ;
#3141=CARTESIAN_POINT ( 'NONE',  ( 44.99999999999999289, 50.00000000000000000, -10.00000000000000533 ) ) ;
#3151=FACE_OUTER_BOUND ( 'NONE', #1883, .T. ) ;
#3154=VERTEX_POINT ( 'NONE', #1755 ) ;
#3157=AXIS2_PLACEMENT_3D ( 'NONE', #2413, #300, #2637 ) ;
#3161=AXIS2_PLACEMENT_3D ( 'NONE', #1485, #1251, #172 ) ;
#3163=AXIS2_PLACEMENT_3D ( 'NONE', #2098, #1046, #2335 ) ;
#3169=ORIENTED_EDGE ( 'NONE', *, *, #1869, .F. ) ;
#3174=VERTEX_POINT ( 'NONE', #642 ) ;
#3175=DIRECTION ( 'NONE',  ( -0.000000000000000000, 1.000000000000000000, -0.000000000000000000 ) ) ;
#3177=ORIENTED_EDGE ( 'NONE', *, *, #2595, .F. ) ;
#3179=FILL_AREA_STYLE ('',( #2912 ) ) ;
#3182=EDGE_CURVE ( 'NONE', #1968, #1875, #2727, .T. ) ;
#3185=EDGE_LOOP ( 'NONE', ( #1594, #1478, #192, #381 ) ) ;
#3189=LINE ( 'NONE', #2127, #921 ) ;
#3190=VERTEX_POINT ( 'NONE', #690 ) ;
#3191=ADVANCED_FACE ( 'NONE', ( #393 ), #1974, .T. ) ;
#3198=ORIENTED_EDGE ( 'NONE', *, *, #630, .F. ) ;
#3200=PLANE ( 'NONE',  #2500 ) ;
#3201=EDGE_LOOP ( 'NONE', ( #655, #2946 ) ) ;
#3203=VERTEX_POINT ( 'NONE', #2754 ) ;
#3204=FACE_OUTER_BOUND ( 'NONE', #2704, .T. ) ;
#3206=EDGE_CURVE ( 'NONE', #895, #499, #2282, .T. ) ;
#3207=DIRECTION ( 'NONE',  ( 0.000000000000000000, 0.000000000000000000, 1.000000000000000000 ) ) ;
#3208=CONICAL_SURFACE ( 'NONE', #965, 2.000000000000001776, 1.029744258676657642 ) ;
#3209=CARTESIAN_POINT ( 'NONE',  ( -44.99999999999999289, 45.00000000000000711, 12.00000000000000711 ) ) ;
#3210=CARTESIAN_POINT ( 'NONE',  ( 66.99999999999997158, -5.000000000000000000, 41.99999999999999289 ) ) ;
#3213=EDGE_CURVE ( 'NONE', #3026, #121, #954, .T. ) ;
#3215=VERTEX_POINT ( 'NONE', #1482 ) ;
#3216=CONICAL_SURFACE ( 'NONE', #2176, 2.000000000000001776, 1.029744258676657642 ) ;
#3219=CARTESIAN_POINT ( 'NONE',  ( 66.99999999999997158, -5.000000000000000000, 44.49999999999999289 ) ) ;
#3221=VECTOR ( 'NONE', #3266, 1000.000000000000000 ) ;
#3222=DIRECTION ( 'NONE',  ( -0.000000000000000000, 1.000000000000000000, -0.000000000000000000 ) ) ;
#3230=DIRECTION ( 'NONE',  ( 0.000000000000000000, 0.000000000000000000, 1.000000000000000000 ) ) ;
#3233=CARTESIAN_POINT ( 'NONE',  ( -44.99999999999999289, 45.00000000000000711, 10.00000000000000533 ) ) ;
#3237=EDGE_CURVE ( 'NONE', #2972, #594, #968, .T. ) ;
#3238=CARTESIAN_POINT ( 'NONE',  ( -44.99999999999999289, 50.00000000000000000, 10.00000000000000533 ) ) ;
#3241=CARTESIAN_POINT ( 'NONE',  ( -75.00000000000000000, 0.000000000000000000, 50.00000000000000000 ) ) ;
#3247=FACE_OUTER_BOUND ( 'NONE', #1726, .T. ) ;
#3251=DIRECTION ( 'NONE',  ( 0.000000000000000000, 0.000000000000000000, 1.000000000000000000 ) ) ;
#3254=ORIENTED_EDGE ( 'NONE', *, *, #2132, .F. ) ;
#3258=EDGE_LOOP ( 'NONE', ( #2380, #372, #1911, #180 ) ) ;
#3261=DIRECTION ( 'NONE',  ( 0.000000000000000000, 0.000000000000000000, 1.000000000000000000 ) ) ;
#3266=DIRECTION ( 'NONE',  ( -1.000000000000000000, -0.000000000000000000, -0.000000000000000000 ) ) ;
#3269=AXIS2_PLACEMENT_3D ( 'NONE', #65, #1599, #2926 ) ;
#3274=STYLED_ITEM('',(#3415),#2792);
#3282=CYLINDRICAL_SURFACE ( 'NONE', #2490, 2.000000000000001776 ) ;
#3285=CARTESIAN_POINT ( 'NONE',  ( -44.99999999999999289, 45.00000000000000711, 10.00000000000000533 ) ) ;
#3286=EDGE_LOOP ( 'NONE', ( #3082, #2756, #828, #2955 ) ) ;
#3296=DIRECTION ( 'NONE',  ( 0.000000000000000000, -1.000000000000000000, 0.000000000000000000 ) ) ;
#3297=DIRECTION ( 'NONE',  ( -0.000000000000000000, 1.000000000000000000, -0.000000000000000000 ) ) ;
#3299=CARTESIAN_POINT ( 'NONE',  ( -74.99999999999998579, 50.00000000000000000, -50.00000000000000000 ) ) ;
#3303=PLANE ( 'NONE',  #1353 ) ;
#3308=ORIENTED_EDGE ( 'NONE', *, *, #3237, .F. ) ;
#3315=ADVANCED_FACE ( 'NONE', ( #507 ), #270, .F. ) ;
#3318=AXIS2_PLACEMENT_3D ( 'NONE', #937, #883, #660 ) ;
#3322=CIRCLE ( 'NONE', #1194, 2.000000000000001776 ) ;
#3324=ORIENTED_EDGE ( 'NONE', *, *, #2652, .F. ) ;
#3325=AXIS2_PLACEMENT_3D ( 'NONE', #1110, #2346, #552 ) ;
#3330=CIRCLE ( 'NONE', #55, 2.499999999999995115 ) ;
#3332=ORIENTED_EDGE ( 'NONE', *, *, #842, .T. ) ;
#3339=ADVANCED_FACE ( 'NONE', ( #2095 ), #2075, .F. ) ;
#3342=DIRECTION ( 'NONE',  ( -0.000000000000000000, 1.000000000000000000, -0.000000000000000000 ) ) ;
#3348=LINE ( 'NONE', #1241, #1086 ) ;
#3351=DIRECTION ( 'NONE',  ( 0.000000000000000000, -1.000000000000000000, 0.000000000000000000 ) ) ;
#3355=ORIENTED_EDGE ( 'NONE', *, *, #24, .T. ) ;
#3359=EDGE_LOOP ( 'NONE', ( #2155, #176, #307, #1374 ) ) ;
#3360=DIRECTION ( 'NONE',  ( 0.000000000000000000, -1.000000000000000000, 0.000000000000000000 ) ) ;
#3372=DIRECTION ( 'NONE',  ( 1.000000000000000000, 0.000000000000000000, -0.000000000000000000 ) ) ;
#3409=COLOUR_RGB('Grey',0.48,0.52,0.57);
#3410=FILL_AREA_STYLE_COLOUR('',#3409);
#3411=FILL_AREA_STYLE('',(#3410));
#3412=SURFACE_STYLE_FILL_AREA(#3411);
#3413=SURFACE_SIDE_STYLE('',(#3412));
#3414=SURFACE_STYLE_USAGE(.BOTH.,#3413);
#3415=PRESENTATION_STYLE_ASSIGNMENT((#3414));
ENDSEC;
END-ISO-10303-21;
